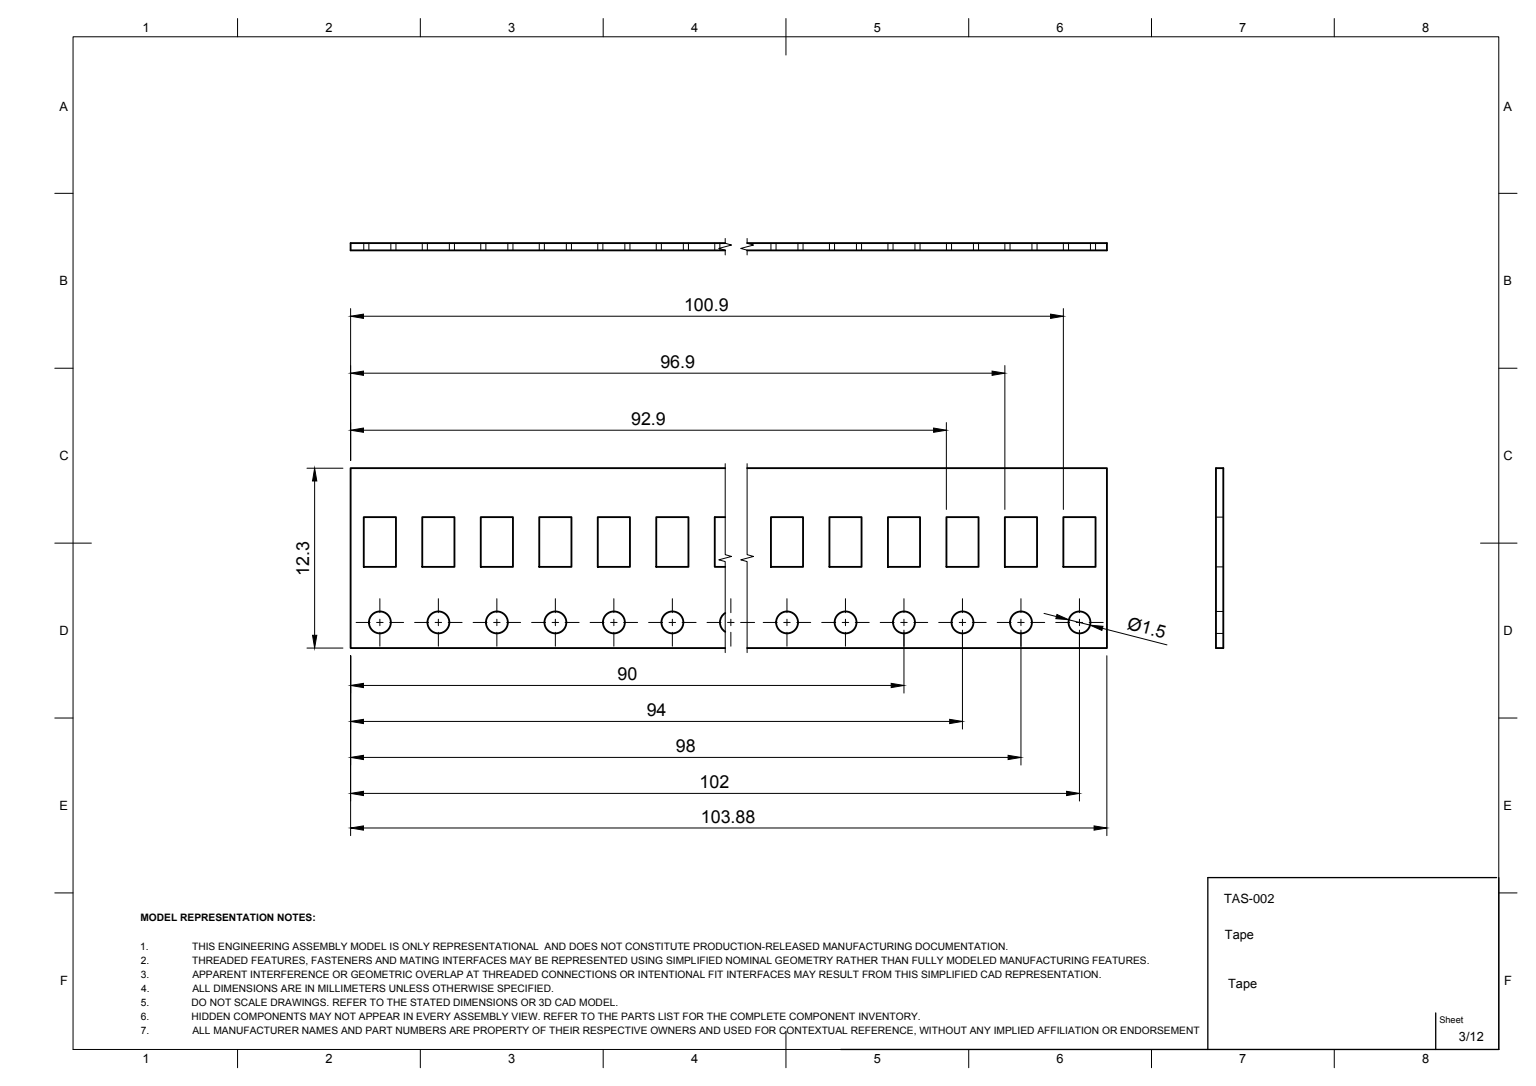
ISO-10303-21;
HEADER;
/* Generated by software containing ST-Developer
 * from STEP Tools, Inc. (www.steptools.com) 
 */

FILE_DESCRIPTION(
/* description */ ('STEP AP214'),
/* implementation_level */ '2;1');

FILE_NAME(
/* name */ 'Tape.step',
/* time_stamp */ '2026-11-04T19:38:14-08:00',
/* author */ (''),
/* organization */ (''),
/* preprocessor_version */ 'ST-DEVELOPER v20.2',
/* originating_system */ 'Autodesk Translation Framework v15.17.0.0',
/* authorisation */ '');

FILE_SCHEMA (('AUTOMOTIVE_DESIGN { 1 0 10303 214 3 1 1 }'));
ENDSEC;

DATA;
#10=MECHANICAL_DESIGN_GEOMETRIC_PRESENTATION_REPRESENTATION('',(#470),#36668);
#450=SHAPE_REPRESENTATION_RELATIONSHIP('SRR','None',#36706,#460);
#460=ADVANCED_BREP_SHAPE_REPRESENTATION('',(#480),#36658);
#470=STYLED_ITEM('',(#36765),#480);
#480=MANIFOLD_SOLID_BREP('Body1',#17793);
#489=CYLINDRICAL_SURFACE('',#17972,0.750000000000001);
#490=CYLINDRICAL_SURFACE('',#17973,0.750000000000001);
#491=CYLINDRICAL_SURFACE('',#17974,0.75);
#492=CYLINDRICAL_SURFACE('',#17975,0.75);
#493=CYLINDRICAL_SURFACE('',#17976,0.75);
#494=CYLINDRICAL_SURFACE('',#17977,0.75);
#495=CYLINDRICAL_SURFACE('',#17978,0.750000000000001);
#496=CYLINDRICAL_SURFACE('',#17979,0.750000000000001);
#497=CYLINDRICAL_SURFACE('',#17980,0.750000000000001);
#498=CYLINDRICAL_SURFACE('',#17981,0.750000000000001);
#499=CYLINDRICAL_SURFACE('',#17982,0.750000000000001);
#500=CYLINDRICAL_SURFACE('',#17983,0.750000000000001);
#501=CYLINDRICAL_SURFACE('',#17984,0.750000000000001);
#502=CYLINDRICAL_SURFACE('',#17985,0.750000000000001);
#503=CYLINDRICAL_SURFACE('',#17986,0.750000000000001);
#504=CYLINDRICAL_SURFACE('',#17987,0.750000000000001);
#505=CYLINDRICAL_SURFACE('',#17988,0.750000000000001);
#506=CYLINDRICAL_SURFACE('',#17989,0.750000000000001);
#507=CYLINDRICAL_SURFACE('',#17990,0.750000000000001);
#508=CYLINDRICAL_SURFACE('',#17991,0.750000000000001);
#509=CYLINDRICAL_SURFACE('',#17992,0.750000000000001);
#510=CYLINDRICAL_SURFACE('',#17993,0.750000000000001);
#511=CYLINDRICAL_SURFACE('',#17994,0.750000000000001);
#512=CYLINDRICAL_SURFACE('',#17995,0.750000000000001);
#513=CYLINDRICAL_SURFACE('',#17996,0.750000000000001);
#514=CYLINDRICAL_SURFACE('',#17997,0.750000000000001);
#776=FACE_BOUND('',#2459,.T.);
#777=FACE_BOUND('',#2460,.T.);
#778=FACE_BOUND('',#2461,.T.);
#779=FACE_BOUND('',#2462,.T.);
#780=FACE_BOUND('',#2463,.T.);
#781=FACE_BOUND('',#2464,.T.);
#782=FACE_BOUND('',#2465,.T.);
#783=FACE_BOUND('',#2466,.T.);
#784=FACE_BOUND('',#2467,.T.);
#785=FACE_BOUND('',#2468,.T.);
#786=FACE_BOUND('',#2469,.T.);
#787=FACE_BOUND('',#2470,.T.);
#788=FACE_BOUND('',#2471,.T.);
#789=FACE_BOUND('',#2472,.T.);
#790=FACE_BOUND('',#2473,.T.);
#791=FACE_BOUND('',#2474,.T.);
#792=FACE_BOUND('',#2475,.T.);
#793=FACE_BOUND('',#2476,.T.);
#794=FACE_BOUND('',#2477,.T.);
#795=FACE_BOUND('',#2478,.T.);
#796=FACE_BOUND('',#2479,.T.);
#797=FACE_BOUND('',#2480,.T.);
#798=FACE_BOUND('',#2481,.T.);
#799=FACE_BOUND('',#2482,.T.);
#800=FACE_BOUND('',#2483,.T.);
#801=FACE_BOUND('',#2484,.T.);
#802=FACE_BOUND('',#2485,.T.);
#803=FACE_BOUND('',#2486,.T.);
#804=FACE_BOUND('',#2487,.T.);
#805=FACE_BOUND('',#2488,.T.);
#806=FACE_BOUND('',#2489,.T.);
#807=FACE_BOUND('',#2490,.T.);
#808=FACE_BOUND('',#2491,.T.);
#809=FACE_BOUND('',#2492,.T.);
#810=FACE_BOUND('',#2493,.T.);
#811=FACE_BOUND('',#2494,.T.);
#812=FACE_BOUND('',#2495,.T.);
#813=FACE_BOUND('',#2496,.T.);
#814=FACE_BOUND('',#2497,.T.);
#815=FACE_BOUND('',#2498,.T.);
#816=FACE_BOUND('',#2499,.T.);
#817=FACE_BOUND('',#2500,.T.);
#818=FACE_BOUND('',#2501,.T.);
#819=FACE_BOUND('',#2502,.T.);
#820=FACE_BOUND('',#2503,.T.);
#821=FACE_BOUND('',#2504,.T.);
#822=FACE_BOUND('',#2505,.T.);
#823=FACE_BOUND('',#2506,.T.);
#824=FACE_BOUND('',#2507,.T.);
#825=FACE_BOUND('',#2508,.T.);
#826=FACE_BOUND('',#2509,.T.);
#827=FACE_BOUND('',#2510,.T.);
#828=FACE_BOUND('',#2512,.T.);
#829=FACE_BOUND('',#2513,.T.);
#830=FACE_BOUND('',#2514,.T.);
#831=FACE_BOUND('',#2515,.T.);
#832=FACE_BOUND('',#2516,.T.);
#833=FACE_BOUND('',#2517,.T.);
#834=FACE_BOUND('',#2518,.T.);
#835=FACE_BOUND('',#2519,.T.);
#836=FACE_BOUND('',#2520,.T.);
#837=FACE_BOUND('',#2521,.T.);
#838=FACE_BOUND('',#2522,.T.);
#839=FACE_BOUND('',#2523,.T.);
#840=FACE_BOUND('',#2524,.T.);
#841=FACE_BOUND('',#2525,.T.);
#842=FACE_BOUND('',#2526,.T.);
#843=FACE_BOUND('',#2527,.T.);
#844=FACE_BOUND('',#2528,.T.);
#845=FACE_BOUND('',#2529,.T.);
#846=FACE_BOUND('',#2530,.T.);
#847=FACE_BOUND('',#2531,.T.);
#848=FACE_BOUND('',#2532,.T.);
#849=FACE_BOUND('',#2533,.T.);
#850=FACE_BOUND('',#2534,.T.);
#851=FACE_BOUND('',#2535,.T.);
#852=FACE_BOUND('',#2536,.T.);
#853=FACE_BOUND('',#2537,.T.);
#854=FACE_BOUND('',#2538,.T.);
#855=FACE_BOUND('',#2539,.T.);
#856=FACE_BOUND('',#2540,.T.);
#857=FACE_BOUND('',#2541,.T.);
#858=FACE_BOUND('',#2542,.T.);
#859=FACE_BOUND('',#2543,.T.);
#860=FACE_BOUND('',#2544,.T.);
#861=FACE_BOUND('',#2545,.T.);
#862=FACE_BOUND('',#2546,.T.);
#863=FACE_BOUND('',#2547,.T.);
#864=FACE_BOUND('',#2548,.T.);
#865=FACE_BOUND('',#2549,.T.);
#866=FACE_BOUND('',#2550,.T.);
#867=FACE_BOUND('',#2551,.T.);
#868=FACE_BOUND('',#2552,.T.);
#869=FACE_BOUND('',#2553,.T.);
#870=FACE_BOUND('',#2554,.T.);
#871=FACE_BOUND('',#2555,.T.);
#872=FACE_BOUND('',#2556,.T.);
#873=FACE_BOUND('',#2557,.T.);
#874=FACE_BOUND('',#2558,.T.);
#875=FACE_BOUND('',#2559,.T.);
#876=FACE_BOUND('',#2560,.T.);
#877=FACE_BOUND('',#2561,.T.);
#878=FACE_BOUND('',#2562,.T.);
#879=FACE_BOUND('',#2563,.T.);
#973=CIRCLE('',#17918,0.750000000000001);
#974=CIRCLE('',#17919,0.750000000000001);
#975=CIRCLE('',#17920,0.750000000000001);
#976=CIRCLE('',#17921,0.75);
#977=CIRCLE('',#17922,0.75);
#978=CIRCLE('',#17923,0.75);
#979=CIRCLE('',#17924,0.75);
#980=CIRCLE('',#17925,0.750000000000001);
#981=CIRCLE('',#17926,0.750000000000001);
#982=CIRCLE('',#17927,0.750000000000001);
#983=CIRCLE('',#17928,0.750000000000001);
#984=CIRCLE('',#17929,0.750000000000001);
#985=CIRCLE('',#17930,0.750000000000001);
#986=CIRCLE('',#17931,0.750000000000001);
#987=CIRCLE('',#17932,0.750000000000001);
#988=CIRCLE('',#17933,0.750000000000001);
#989=CIRCLE('',#17934,0.750000000000001);
#990=CIRCLE('',#17935,0.750000000000001);
#991=CIRCLE('',#17936,0.750000000000001);
#992=CIRCLE('',#17937,0.750000000000001);
#993=CIRCLE('',#17938,0.750000000000001);
#994=CIRCLE('',#17939,0.750000000000001);
#995=CIRCLE('',#17940,0.750000000000001);
#996=CIRCLE('',#17941,0.750000000000001);
#997=CIRCLE('',#17942,0.750000000000001);
#998=CIRCLE('',#17943,0.750000000000001);
#999=CIRCLE('',#17945,0.750000000000001);
#1000=CIRCLE('',#17946,0.750000000000001);
#1001=CIRCLE('',#17947,0.750000000000001);
#1002=CIRCLE('',#17948,0.750000000000001);
#1003=CIRCLE('',#17949,0.750000000000001);
#1004=CIRCLE('',#17950,0.750000000000001);
#1005=CIRCLE('',#17951,0.750000000000001);
#1006=CIRCLE('',#17952,0.750000000000001);
#1007=CIRCLE('',#17953,0.750000000000001);
#1008=CIRCLE('',#17954,0.750000000000001);
#1009=CIRCLE('',#17955,0.750000000000001);
#1010=CIRCLE('',#17956,0.750000000000001);
#1011=CIRCLE('',#17957,0.750000000000001);
#1012=CIRCLE('',#17958,0.750000000000001);
#1013=CIRCLE('',#17959,0.750000000000001);
#1014=CIRCLE('',#17960,0.750000000000001);
#1015=CIRCLE('',#17961,0.750000000000001);
#1016=CIRCLE('',#17962,0.750000000000001);
#1017=CIRCLE('',#17963,0.750000000000001);
#1018=CIRCLE('',#17964,0.75);
#1019=CIRCLE('',#17965,0.75);
#1020=CIRCLE('',#17966,0.75);
#1021=CIRCLE('',#17967,0.75);
#1022=CIRCLE('',#17968,0.750000000000001);
#1023=CIRCLE('',#17969,0.750000000000001);
#1024=CIRCLE('',#17970,0.750000000000001);
#1527=FACE_OUTER_BOUND('',#2458,.T.);
#1528=FACE_OUTER_BOUND('',#2511,.T.);
#1529=FACE_OUTER_BOUND('',#2564,.T.);
#1530=FACE_OUTER_BOUND('',#2565,.T.);
#1531=FACE_OUTER_BOUND('',#2566,.T.);
#1532=FACE_OUTER_BOUND('',#2567,.T.);
#1533=FACE_OUTER_BOUND('',#2568,.T.);
#1534=FACE_OUTER_BOUND('',#2569,.T.);
#1535=FACE_OUTER_BOUND('',#2570,.T.);
#1536=FACE_OUTER_BOUND('',#2571,.T.);
#1537=FACE_OUTER_BOUND('',#2572,.T.);
#1538=FACE_OUTER_BOUND('',#2573,.T.);
#1539=FACE_OUTER_BOUND('',#2574,.T.);
#1540=FACE_OUTER_BOUND('',#2575,.T.);
#1541=FACE_OUTER_BOUND('',#2576,.T.);
#1542=FACE_OUTER_BOUND('',#2577,.T.);
#1543=FACE_OUTER_BOUND('',#2578,.T.);
#1544=FACE_OUTER_BOUND('',#2579,.T.);
#1545=FACE_OUTER_BOUND('',#2580,.T.);
#1546=FACE_OUTER_BOUND('',#2581,.T.);
#1547=FACE_OUTER_BOUND('',#2582,.T.);
#1548=FACE_OUTER_BOUND('',#2583,.T.);
#1549=FACE_OUTER_BOUND('',#2584,.T.);
#1550=FACE_OUTER_BOUND('',#2585,.T.);
#1551=FACE_OUTER_BOUND('',#2586,.T.);
#1552=FACE_OUTER_BOUND('',#2587,.T.);
#1553=FACE_OUTER_BOUND('',#2588,.T.);
#1554=FACE_OUTER_BOUND('',#2589,.T.);
#1555=FACE_OUTER_BOUND('',#2590,.T.);
#1556=FACE_OUTER_BOUND('',#2591,.T.);
#1557=FACE_OUTER_BOUND('',#2592,.T.);
#1558=FACE_OUTER_BOUND('',#2593,.T.);
#1559=FACE_OUTER_BOUND('',#2594,.T.);
#1560=FACE_OUTER_BOUND('',#2595,.T.);
#1561=FACE_OUTER_BOUND('',#2596,.T.);
#1562=FACE_OUTER_BOUND('',#2597,.T.);
#1563=FACE_OUTER_BOUND('',#2598,.T.);
#1564=FACE_OUTER_BOUND('',#2599,.T.);
#1565=FACE_OUTER_BOUND('',#2600,.T.);
#1566=FACE_OUTER_BOUND('',#2601,.T.);
#1567=FACE_OUTER_BOUND('',#2602,.T.);
#1568=FACE_OUTER_BOUND('',#2603,.T.);
#1569=FACE_OUTER_BOUND('',#2604,.T.);
#1570=FACE_OUTER_BOUND('',#2605,.T.);
#1571=FACE_OUTER_BOUND('',#2606,.T.);
#1572=FACE_OUTER_BOUND('',#2607,.T.);
#1573=FACE_OUTER_BOUND('',#2608,.T.);
#1574=FACE_OUTER_BOUND('',#2609,.T.);
#1575=FACE_OUTER_BOUND('',#2610,.T.);
#1576=FACE_OUTER_BOUND('',#2611,.T.);
#1577=FACE_OUTER_BOUND('',#2612,.T.);
#1578=FACE_OUTER_BOUND('',#2613,.T.);
#1579=FACE_OUTER_BOUND('',#2614,.T.);
#1580=FACE_OUTER_BOUND('',#2615,.T.);
#1581=FACE_OUTER_BOUND('',#2616,.T.);
#1582=FACE_OUTER_BOUND('',#2617,.T.);
#1583=FACE_OUTER_BOUND('',#2618,.T.);
#1584=FACE_OUTER_BOUND('',#2619,.T.);
#1585=FACE_OUTER_BOUND('',#2620,.T.);
#1586=FACE_OUTER_BOUND('',#2621,.T.);
#1587=FACE_OUTER_BOUND('',#2622,.T.);
#1588=FACE_OUTER_BOUND('',#2623,.T.);
#1589=FACE_OUTER_BOUND('',#2624,.T.);
#1590=FACE_OUTER_BOUND('',#2625,.T.);
#1591=FACE_OUTER_BOUND('',#2626,.T.);
#1592=FACE_OUTER_BOUND('',#2627,.T.);
#1593=FACE_OUTER_BOUND('',#2628,.T.);
#1594=FACE_OUTER_BOUND('',#2629,.T.);
#1595=FACE_OUTER_BOUND('',#2630,.T.);
#1596=FACE_OUTER_BOUND('',#2631,.T.);
#1597=FACE_OUTER_BOUND('',#2632,.T.);
#1598=FACE_OUTER_BOUND('',#2633,.T.);
#1599=FACE_OUTER_BOUND('',#2634,.T.);
#1600=FACE_OUTER_BOUND('',#2635,.T.);
#1601=FACE_OUTER_BOUND('',#2636,.T.);
#1602=FACE_OUTER_BOUND('',#2637,.T.);
#1603=FACE_OUTER_BOUND('',#2638,.T.);
#1604=FACE_OUTER_BOUND('',#2639,.T.);
#1605=FACE_OUTER_BOUND('',#2640,.T.);
#1606=FACE_OUTER_BOUND('',#2641,.T.);
#1607=FACE_OUTER_BOUND('',#2642,.T.);
#1608=FACE_OUTER_BOUND('',#2643,.T.);
#1609=FACE_OUTER_BOUND('',#2644,.T.);
#1610=FACE_OUTER_BOUND('',#2645,.T.);
#1611=FACE_OUTER_BOUND('',#2646,.T.);
#1612=FACE_OUTER_BOUND('',#2647,.T.);
#1613=FACE_OUTER_BOUND('',#2648,.T.);
#1614=FACE_OUTER_BOUND('',#2649,.T.);
#1615=FACE_OUTER_BOUND('',#2650,.T.);
#1616=FACE_OUTER_BOUND('',#2651,.T.);
#1617=FACE_OUTER_BOUND('',#2652,.T.);
#1618=FACE_OUTER_BOUND('',#2653,.T.);
#1619=FACE_OUTER_BOUND('',#2654,.T.);
#1620=FACE_OUTER_BOUND('',#2655,.T.);
#1621=FACE_OUTER_BOUND('',#2656,.T.);
#1622=FACE_OUTER_BOUND('',#2657,.T.);
#1623=FACE_OUTER_BOUND('',#2658,.T.);
#1624=FACE_OUTER_BOUND('',#2659,.T.);
#1625=FACE_OUTER_BOUND('',#2660,.T.);
#1626=FACE_OUTER_BOUND('',#2661,.T.);
#1627=FACE_OUTER_BOUND('',#2662,.T.);
#1628=FACE_OUTER_BOUND('',#2663,.T.);
#1629=FACE_OUTER_BOUND('',#2664,.T.);
#1630=FACE_OUTER_BOUND('',#2665,.T.);
#1631=FACE_OUTER_BOUND('',#2666,.T.);
#1632=FACE_OUTER_BOUND('',#2667,.T.);
#1633=FACE_OUTER_BOUND('',#2668,.T.);
#1634=FACE_OUTER_BOUND('',#2669,.T.);
#1635=FACE_OUTER_BOUND('',#2670,.T.);
#1636=FACE_OUTER_BOUND('',#2671,.T.);
#1637=FACE_OUTER_BOUND('',#2672,.T.);
#1638=FACE_OUTER_BOUND('',#2673,.T.);
#1639=FACE_OUTER_BOUND('',#2674,.T.);
#1640=FACE_OUTER_BOUND('',#2675,.T.);
#1641=FACE_OUTER_BOUND('',#2676,.T.);
#1642=FACE_OUTER_BOUND('',#2677,.T.);
#1643=FACE_OUTER_BOUND('',#2678,.T.);
#1644=FACE_OUTER_BOUND('',#2679,.T.);
#1645=FACE_OUTER_BOUND('',#2680,.T.);
#1646=FACE_OUTER_BOUND('',#2681,.T.);
#1647=FACE_OUTER_BOUND('',#2682,.T.);
#1648=FACE_OUTER_BOUND('',#2683,.T.);
#1649=FACE_OUTER_BOUND('',#2684,.T.);
#1650=FACE_OUTER_BOUND('',#2685,.T.);
#1651=FACE_OUTER_BOUND('',#2686,.T.);
#1652=FACE_OUTER_BOUND('',#2687,.T.);
#1653=FACE_OUTER_BOUND('',#2688,.T.);
#1654=FACE_OUTER_BOUND('',#2689,.T.);
#1655=FACE_OUTER_BOUND('',#2690,.T.);
#1656=FACE_OUTER_BOUND('',#2691,.T.);
#1657=FACE_OUTER_BOUND('',#2692,.T.);
#1658=FACE_OUTER_BOUND('',#2693,.T.);
#1659=FACE_OUTER_BOUND('',#2694,.T.);
#1660=FACE_OUTER_BOUND('',#2695,.T.);
#1661=FACE_OUTER_BOUND('',#2696,.T.);
#1662=FACE_OUTER_BOUND('',#2697,.T.);
#2458=EDGE_LOOP('',(#11214,#11215,#11216,#11217));
#2459=EDGE_LOOP('',(#11218));
#2460=EDGE_LOOP('',(#11219));
#2461=EDGE_LOOP('',(#11220));
#2462=EDGE_LOOP('',(#11221));
#2463=EDGE_LOOP('',(#11222));
#2464=EDGE_LOOP('',(#11223));
#2465=EDGE_LOOP('',(#11224));
#2466=EDGE_LOOP('',(#11225));
#2467=EDGE_LOOP('',(#11226));
#2468=EDGE_LOOP('',(#11227));
#2469=EDGE_LOOP('',(#11228));
#2470=EDGE_LOOP('',(#11229));
#2471=EDGE_LOOP('',(#11230));
#2472=EDGE_LOOP('',(#11231));
#2473=EDGE_LOOP('',(#11232));
#2474=EDGE_LOOP('',(#11233));
#2475=EDGE_LOOP('',(#11234));
#2476=EDGE_LOOP('',(#11235));
#2477=EDGE_LOOP('',(#11236));
#2478=EDGE_LOOP('',(#11237));
#2479=EDGE_LOOP('',(#11238));
#2480=EDGE_LOOP('',(#11239));
#2481=EDGE_LOOP('',(#11240));
#2482=EDGE_LOOP('',(#11241));
#2483=EDGE_LOOP('',(#11242));
#2484=EDGE_LOOP('',(#11243));
#2485=EDGE_LOOP('',(#11244,#11245,#11246,#11247));
#2486=EDGE_LOOP('',(#11248,#11249,#11250,#11251));
#2487=EDGE_LOOP('',(#11252,#11253,#11254,#11255));
#2488=EDGE_LOOP('',(#11256,#11257,#11258,#11259));
#2489=EDGE_LOOP('',(#11260,#11261,#11262,#11263));
#2490=EDGE_LOOP('',(#11264,#11265,#11266,#11267));
#2491=EDGE_LOOP('',(#11268,#11269,#11270,#11271));
#2492=EDGE_LOOP('',(#11272,#11273,#11274,#11275));
#2493=EDGE_LOOP('',(#11276,#11277,#11278,#11279));
#2494=EDGE_LOOP('',(#11280,#11281,#11282,#11283));
#2495=EDGE_LOOP('',(#11284,#11285,#11286,#11287));
#2496=EDGE_LOOP('',(#11288,#11289,#11290,#11291));
#2497=EDGE_LOOP('',(#11292,#11293,#11294,#11295));
#2498=EDGE_LOOP('',(#11296,#11297,#11298,#11299));
#2499=EDGE_LOOP('',(#11300,#11301,#11302,#11303));
#2500=EDGE_LOOP('',(#11304,#11305,#11306,#11307));
#2501=EDGE_LOOP('',(#11308,#11309,#11310,#11311));
#2502=EDGE_LOOP('',(#11312,#11313,#11314,#11315));
#2503=EDGE_LOOP('',(#11316,#11317,#11318,#11319));
#2504=EDGE_LOOP('',(#11320,#11321,#11322,#11323));
#2505=EDGE_LOOP('',(#11324,#11325,#11326,#11327));
#2506=EDGE_LOOP('',(#11328,#11329,#11330,#11331));
#2507=EDGE_LOOP('',(#11332,#11333,#11334,#11335));
#2508=EDGE_LOOP('',(#11336,#11337,#11338,#11339));
#2509=EDGE_LOOP('',(#11340,#11341,#11342,#11343));
#2510=EDGE_LOOP('',(#11344,#11345,#11346,#11347));
#2511=EDGE_LOOP('',(#11348,#11349,#11350,#11351));
#2512=EDGE_LOOP('',(#11352,#11353,#11354,#11355));
#2513=EDGE_LOOP('',(#11356,#11357,#11358,#11359));
#2514=EDGE_LOOP('',(#11360,#11361,#11362,#11363));
#2515=EDGE_LOOP('',(#11364,#11365,#11366,#11367));
#2516=EDGE_LOOP('',(#11368,#11369,#11370,#11371));
#2517=EDGE_LOOP('',(#11372,#11373,#11374,#11375));
#2518=EDGE_LOOP('',(#11376,#11377,#11378,#11379));
#2519=EDGE_LOOP('',(#11380,#11381,#11382,#11383));
#2520=EDGE_LOOP('',(#11384,#11385,#11386,#11387));
#2521=EDGE_LOOP('',(#11388,#11389,#11390,#11391));
#2522=EDGE_LOOP('',(#11392,#11393,#11394,#11395));
#2523=EDGE_LOOP('',(#11396,#11397,#11398,#11399));
#2524=EDGE_LOOP('',(#11400,#11401,#11402,#11403));
#2525=EDGE_LOOP('',(#11404,#11405,#11406,#11407));
#2526=EDGE_LOOP('',(#11408,#11409,#11410,#11411));
#2527=EDGE_LOOP('',(#11412,#11413,#11414,#11415));
#2528=EDGE_LOOP('',(#11416,#11417,#11418,#11419));
#2529=EDGE_LOOP('',(#11420,#11421,#11422,#11423));
#2530=EDGE_LOOP('',(#11424,#11425,#11426,#11427));
#2531=EDGE_LOOP('',(#11428,#11429,#11430,#11431));
#2532=EDGE_LOOP('',(#11432,#11433,#11434,#11435));
#2533=EDGE_LOOP('',(#11436,#11437,#11438,#11439));
#2534=EDGE_LOOP('',(#11440,#11441,#11442,#11443));
#2535=EDGE_LOOP('',(#11444,#11445,#11446,#11447));
#2536=EDGE_LOOP('',(#11448,#11449,#11450,#11451));
#2537=EDGE_LOOP('',(#11452,#11453,#11454,#11455));
#2538=EDGE_LOOP('',(#11456));
#2539=EDGE_LOOP('',(#11457));
#2540=EDGE_LOOP('',(#11458));
#2541=EDGE_LOOP('',(#11459));
#2542=EDGE_LOOP('',(#11460));
#2543=EDGE_LOOP('',(#11461));
#2544=EDGE_LOOP('',(#11462));
#2545=EDGE_LOOP('',(#11463));
#2546=EDGE_LOOP('',(#11464));
#2547=EDGE_LOOP('',(#11465));
#2548=EDGE_LOOP('',(#11466));
#2549=EDGE_LOOP('',(#11467));
#2550=EDGE_LOOP('',(#11468));
#2551=EDGE_LOOP('',(#11469));
#2552=EDGE_LOOP('',(#11470));
#2553=EDGE_LOOP('',(#11471));
#2554=EDGE_LOOP('',(#11472));
#2555=EDGE_LOOP('',(#11473));
#2556=EDGE_LOOP('',(#11474));
#2557=EDGE_LOOP('',(#11475));
#2558=EDGE_LOOP('',(#11476));
#2559=EDGE_LOOP('',(#11477));
#2560=EDGE_LOOP('',(#11478));
#2561=EDGE_LOOP('',(#11479));
#2562=EDGE_LOOP('',(#11480));
#2563=EDGE_LOOP('',(#11481));
#2564=EDGE_LOOP('',(#11482,#11483,#11484,#11485));
#2565=EDGE_LOOP('',(#11486,#11487,#11488,#11489));
#2566=EDGE_LOOP('',(#11490,#11491,#11492,#11493));
#2567=EDGE_LOOP('',(#11494,#11495,#11496,#11497));
#2568=EDGE_LOOP('',(#11498,#11499,#11500,#11501));
#2569=EDGE_LOOP('',(#11502,#11503,#11504,#11505));
#2570=EDGE_LOOP('',(#11506,#11507,#11508,#11509));
#2571=EDGE_LOOP('',(#11510,#11511,#11512,#11513));
#2572=EDGE_LOOP('',(#11514,#11515,#11516,#11517));
#2573=EDGE_LOOP('',(#11518,#11519,#11520,#11521));
#2574=EDGE_LOOP('',(#11522,#11523,#11524,#11525));
#2575=EDGE_LOOP('',(#11526,#11527,#11528,#11529));
#2576=EDGE_LOOP('',(#11530,#11531,#11532,#11533));
#2577=EDGE_LOOP('',(#11534,#11535,#11536,#11537));
#2578=EDGE_LOOP('',(#11538,#11539,#11540,#11541));
#2579=EDGE_LOOP('',(#11542,#11543,#11544,#11545));
#2580=EDGE_LOOP('',(#11546,#11547,#11548,#11549));
#2581=EDGE_LOOP('',(#11550,#11551,#11552,#11553));
#2582=EDGE_LOOP('',(#11554,#11555,#11556,#11557));
#2583=EDGE_LOOP('',(#11558,#11559,#11560,#11561));
#2584=EDGE_LOOP('',(#11562,#11563,#11564,#11565));
#2585=EDGE_LOOP('',(#11566,#11567,#11568,#11569));
#2586=EDGE_LOOP('',(#11570,#11571,#11572,#11573));
#2587=EDGE_LOOP('',(#11574,#11575,#11576,#11577));
#2588=EDGE_LOOP('',(#11578,#11579,#11580,#11581));
#2589=EDGE_LOOP('',(#11582,#11583,#11584,#11585));
#2590=EDGE_LOOP('',(#11586,#11587,#11588,#11589));
#2591=EDGE_LOOP('',(#11590,#11591,#11592,#11593));
#2592=EDGE_LOOP('',(#11594,#11595,#11596,#11597));
#2593=EDGE_LOOP('',(#11598,#11599,#11600,#11601));
#2594=EDGE_LOOP('',(#11602,#11603,#11604,#11605));
#2595=EDGE_LOOP('',(#11606,#11607,#11608,#11609));
#2596=EDGE_LOOP('',(#11610,#11611,#11612,#11613));
#2597=EDGE_LOOP('',(#11614,#11615,#11616,#11617));
#2598=EDGE_LOOP('',(#11618,#11619,#11620,#11621));
#2599=EDGE_LOOP('',(#11622,#11623,#11624,#11625));
#2600=EDGE_LOOP('',(#11626,#11627,#11628,#11629));
#2601=EDGE_LOOP('',(#11630,#11631,#11632,#11633));
#2602=EDGE_LOOP('',(#11634,#11635,#11636,#11637));
#2603=EDGE_LOOP('',(#11638,#11639,#11640,#11641));
#2604=EDGE_LOOP('',(#11642,#11643,#11644,#11645));
#2605=EDGE_LOOP('',(#11646,#11647,#11648,#11649));
#2606=EDGE_LOOP('',(#11650,#11651,#11652,#11653));
#2607=EDGE_LOOP('',(#11654,#11655,#11656,#11657));
#2608=EDGE_LOOP('',(#11658,#11659,#11660,#11661));
#2609=EDGE_LOOP('',(#11662,#11663,#11664,#11665));
#2610=EDGE_LOOP('',(#11666,#11667,#11668,#11669));
#2611=EDGE_LOOP('',(#11670,#11671,#11672,#11673));
#2612=EDGE_LOOP('',(#11674,#11675,#11676,#11677));
#2613=EDGE_LOOP('',(#11678,#11679,#11680,#11681));
#2614=EDGE_LOOP('',(#11682,#11683,#11684,#11685));
#2615=EDGE_LOOP('',(#11686,#11687,#11688,#11689));
#2616=EDGE_LOOP('',(#11690,#11691,#11692,#11693));
#2617=EDGE_LOOP('',(#11694,#11695,#11696,#11697));
#2618=EDGE_LOOP('',(#11698,#11699,#11700,#11701));
#2619=EDGE_LOOP('',(#11702,#11703,#11704,#11705));
#2620=EDGE_LOOP('',(#11706,#11707,#11708,#11709));
#2621=EDGE_LOOP('',(#11710,#11711,#11712,#11713));
#2622=EDGE_LOOP('',(#11714,#11715,#11716,#11717));
#2623=EDGE_LOOP('',(#11718,#11719,#11720,#11721));
#2624=EDGE_LOOP('',(#11722,#11723,#11724,#11725));
#2625=EDGE_LOOP('',(#11726,#11727,#11728,#11729));
#2626=EDGE_LOOP('',(#11730,#11731,#11732,#11733));
#2627=EDGE_LOOP('',(#11734,#11735,#11736,#11737));
#2628=EDGE_LOOP('',(#11738,#11739,#11740,#11741));
#2629=EDGE_LOOP('',(#11742,#11743,#11744,#11745));
#2630=EDGE_LOOP('',(#11746,#11747,#11748,#11749));
#2631=EDGE_LOOP('',(#11750,#11751,#11752,#11753));
#2632=EDGE_LOOP('',(#11754,#11755,#11756,#11757));
#2633=EDGE_LOOP('',(#11758,#11759,#11760,#11761));
#2634=EDGE_LOOP('',(#11762,#11763,#11764,#11765));
#2635=EDGE_LOOP('',(#11766,#11767,#11768,#11769));
#2636=EDGE_LOOP('',(#11770,#11771,#11772,#11773));
#2637=EDGE_LOOP('',(#11774,#11775,#11776,#11777));
#2638=EDGE_LOOP('',(#11778,#11779,#11780,#11781));
#2639=EDGE_LOOP('',(#11782,#11783,#11784,#11785));
#2640=EDGE_LOOP('',(#11786,#11787,#11788,#11789));
#2641=EDGE_LOOP('',(#11790,#11791,#11792,#11793));
#2642=EDGE_LOOP('',(#11794,#11795,#11796,#11797));
#2643=EDGE_LOOP('',(#11798,#11799,#11800,#11801));
#2644=EDGE_LOOP('',(#11802,#11803,#11804,#11805));
#2645=EDGE_LOOP('',(#11806,#11807,#11808,#11809));
#2646=EDGE_LOOP('',(#11810,#11811,#11812,#11813));
#2647=EDGE_LOOP('',(#11814,#11815,#11816,#11817));
#2648=EDGE_LOOP('',(#11818,#11819,#11820,#11821));
#2649=EDGE_LOOP('',(#11822,#11823,#11824,#11825));
#2650=EDGE_LOOP('',(#11826,#11827,#11828,#11829));
#2651=EDGE_LOOP('',(#11830,#11831,#11832,#11833));
#2652=EDGE_LOOP('',(#11834,#11835,#11836,#11837));
#2653=EDGE_LOOP('',(#11838,#11839,#11840,#11841));
#2654=EDGE_LOOP('',(#11842,#11843,#11844,#11845));
#2655=EDGE_LOOP('',(#11846,#11847,#11848,#11849));
#2656=EDGE_LOOP('',(#11850,#11851,#11852,#11853));
#2657=EDGE_LOOP('',(#11854,#11855,#11856,#11857));
#2658=EDGE_LOOP('',(#11858,#11859,#11860,#11861));
#2659=EDGE_LOOP('',(#11862,#11863,#11864,#11865));
#2660=EDGE_LOOP('',(#11866,#11867,#11868,#11869));
#2661=EDGE_LOOP('',(#11870,#11871,#11872,#11873));
#2662=EDGE_LOOP('',(#11874,#11875,#11876,#11877));
#2663=EDGE_LOOP('',(#11878,#11879,#11880,#11881));
#2664=EDGE_LOOP('',(#11882,#11883,#11884,#11885));
#2665=EDGE_LOOP('',(#11886,#11887,#11888,#11889));
#2666=EDGE_LOOP('',(#11890,#11891,#11892,#11893));
#2667=EDGE_LOOP('',(#11894,#11895,#11896,#11897));
#2668=EDGE_LOOP('',(#11898,#11899,#11900,#11901));
#2669=EDGE_LOOP('',(#11902,#11903,#11904,#11905));
#2670=EDGE_LOOP('',(#11906,#11907,#11908,#11909));
#2671=EDGE_LOOP('',(#11910,#11911,#11912,#11913));
#2672=EDGE_LOOP('',(#11914,#11915,#11916,#11917));
#2673=EDGE_LOOP('',(#11918,#11919,#11920,#11921));
#2674=EDGE_LOOP('',(#11922,#11923,#11924,#11925));
#2675=EDGE_LOOP('',(#11926,#11927,#11928,#11929));
#2676=EDGE_LOOP('',(#11930,#11931,#11932,#11933));
#2677=EDGE_LOOP('',(#11934,#11935,#11936,#11937));
#2678=EDGE_LOOP('',(#11938,#11939,#11940,#11941));
#2679=EDGE_LOOP('',(#11942,#11943,#11944,#11945));
#2680=EDGE_LOOP('',(#11946,#11947,#11948,#11949));
#2681=EDGE_LOOP('',(#11950,#11951,#11952,#11953));
#2682=EDGE_LOOP('',(#11954,#11955,#11956,#11957));
#2683=EDGE_LOOP('',(#11958,#11959,#11960,#11961));
#2684=EDGE_LOOP('',(#11962,#11963,#11964,#11965));
#2685=EDGE_LOOP('',(#11966,#11967,#11968,#11969));
#2686=EDGE_LOOP('',(#11970,#11971,#11972,#11973));
#2687=EDGE_LOOP('',(#11974,#11975,#11976,#11977));
#2688=EDGE_LOOP('',(#11978,#11979,#11980,#11981));
#2689=EDGE_LOOP('',(#11982,#11983,#11984,#11985));
#2690=EDGE_LOOP('',(#11986,#11987,#11988,#11989));
#2691=EDGE_LOOP('',(#11990,#11991,#11992,#11993));
#2692=EDGE_LOOP('',(#11994,#11995,#11996,#11997));
#2693=EDGE_LOOP('',(#11998,#11999,#12000,#12001));
#2694=EDGE_LOOP('',(#12002,#12003,#12004,#12005));
#2695=EDGE_LOOP('',(#12006,#12007,#12008,#12009));
#2696=EDGE_LOOP('',(#12010,#12011,#12012,#12013));
#2697=EDGE_LOOP('',(#12014,#12015,#12016,#12017));
#3586=LINE('',#24199,#5296);
#3587=LINE('',#24201,#5297);
#3588=LINE('',#24203,#5298);
#3589=LINE('',#24204,#5299);
#3590=LINE('',#24259,#5300);
#3591=LINE('',#24261,#5301);
#3592=LINE('',#24263,#5302);
#3593=LINE('',#24264,#5303);
#3594=LINE('',#24267,#5304);
#3595=LINE('',#24269,#5305);
#3596=LINE('',#24271,#5306);
#3597=LINE('',#24272,#5307);
#3598=LINE('',#24275,#5308);
#3599=LINE('',#24277,#5309);
#3600=LINE('',#24279,#5310);
#3601=LINE('',#24280,#5311);
#3602=LINE('',#24283,#5312);
#3603=LINE('',#24285,#5313);
#3604=LINE('',#24287,#5314);
#3605=LINE('',#24288,#5315);
#3606=LINE('',#24291,#5316);
#3607=LINE('',#24293,#5317);
#3608=LINE('',#24295,#5318);
#3609=LINE('',#24296,#5319);
#3610=LINE('',#24299,#5320);
#3611=LINE('',#24301,#5321);
#3612=LINE('',#24303,#5322);
#3613=LINE('',#24304,#5323);
#3614=LINE('',#24307,#5324);
#3615=LINE('',#24309,#5325);
#3616=LINE('',#24311,#5326);
#3617=LINE('',#24312,#5327);
#3618=LINE('',#24315,#5328);
#3619=LINE('',#24317,#5329);
#3620=LINE('',#24319,#5330);
#3621=LINE('',#24320,#5331);
#3622=LINE('',#24323,#5332);
#3623=LINE('',#24325,#5333);
#3624=LINE('',#24327,#5334);
#3625=LINE('',#24328,#5335);
#3626=LINE('',#24331,#5336);
#3627=LINE('',#24333,#5337);
#3628=LINE('',#24335,#5338);
#3629=LINE('',#24336,#5339);
#3630=LINE('',#24339,#5340);
#3631=LINE('',#24341,#5341);
#3632=LINE('',#24343,#5342);
#3633=LINE('',#24344,#5343);
#3634=LINE('',#24347,#5344);
#3635=LINE('',#24349,#5345);
#3636=LINE('',#24351,#5346);
#3637=LINE('',#24352,#5347);
#3638=LINE('',#24355,#5348);
#3639=LINE('',#24357,#5349);
#3640=LINE('',#24359,#5350);
#3641=LINE('',#24360,#5351);
#3642=LINE('',#24363,#5352);
#3643=LINE('',#24365,#5353);
#3644=LINE('',#24367,#5354);
#3645=LINE('',#24368,#5355);
#3646=LINE('',#24371,#5356);
#3647=LINE('',#24373,#5357);
#3648=LINE('',#24375,#5358);
#3649=LINE('',#24376,#5359);
#3650=LINE('',#24379,#5360);
#3651=LINE('',#24381,#5361);
#3652=LINE('',#24383,#5362);
#3653=LINE('',#24384,#5363);
#3654=LINE('',#24387,#5364);
#3655=LINE('',#24389,#5365);
#3656=LINE('',#24391,#5366);
#3657=LINE('',#24392,#5367);
#3658=LINE('',#24395,#5368);
#3659=LINE('',#24397,#5369);
#3660=LINE('',#24399,#5370);
#3661=LINE('',#24400,#5371);
#3662=LINE('',#24403,#5372);
#3663=LINE('',#24405,#5373);
#3664=LINE('',#24407,#5374);
#3665=LINE('',#24408,#5375);
#3666=LINE('',#24411,#5376);
#3667=LINE('',#24413,#5377);
#3668=LINE('',#24415,#5378);
#3669=LINE('',#24416,#5379);
#3670=LINE('',#24419,#5380);
#3671=LINE('',#24421,#5381);
#3672=LINE('',#24423,#5382);
#3673=LINE('',#24424,#5383);
#3674=LINE('',#24427,#5384);
#3675=LINE('',#24429,#5385);
#3676=LINE('',#24431,#5386);
#3677=LINE('',#24432,#5387);
#3678=LINE('',#24435,#5388);
#3679=LINE('',#24437,#5389);
#3680=LINE('',#24439,#5390);
#3681=LINE('',#24440,#5391);
#3682=LINE('',#24443,#5392);
#3683=LINE('',#24445,#5393);
#3684=LINE('',#24447,#5394);
#3685=LINE('',#24448,#5395);
#3686=LINE('',#24451,#5396);
#3687=LINE('',#24453,#5397);
#3688=LINE('',#24455,#5398);
#3689=LINE('',#24456,#5399);
#3690=LINE('',#24459,#5400);
#3691=LINE('',#24461,#5401);
#3692=LINE('',#24463,#5402);
#3693=LINE('',#24464,#5403);
#3694=LINE('',#24468,#5404);
#3695=LINE('',#24470,#5405);
#3696=LINE('',#24472,#5406);
#3697=LINE('',#24473,#5407);
#3698=LINE('',#24476,#5408);
#3699=LINE('',#24478,#5409);
#3700=LINE('',#24480,#5410);
#3701=LINE('',#24481,#5411);
#3702=LINE('',#24484,#5412);
#3703=LINE('',#24486,#5413);
#3704=LINE('',#24488,#5414);
#3705=LINE('',#24489,#5415);
#3706=LINE('',#24492,#5416);
#3707=LINE('',#24494,#5417);
#3708=LINE('',#24496,#5418);
#3709=LINE('',#24497,#5419);
#3710=LINE('',#24500,#5420);
#3711=LINE('',#24502,#5421);
#3712=LINE('',#24504,#5422);
#3713=LINE('',#24505,#5423);
#3714=LINE('',#24508,#5424);
#3715=LINE('',#24510,#5425);
#3716=LINE('',#24512,#5426);
#3717=LINE('',#24513,#5427);
#3718=LINE('',#24516,#5428);
#3719=LINE('',#24518,#5429);
#3720=LINE('',#24520,#5430);
#3721=LINE('',#24521,#5431);
#3722=LINE('',#24524,#5432);
#3723=LINE('',#24526,#5433);
#3724=LINE('',#24528,#5434);
#3725=LINE('',#24529,#5435);
#3726=LINE('',#24532,#5436);
#3727=LINE('',#24534,#5437);
#3728=LINE('',#24536,#5438);
#3729=LINE('',#24537,#5439);
#3730=LINE('',#24540,#5440);
#3731=LINE('',#24542,#5441);
#3732=LINE('',#24544,#5442);
#3733=LINE('',#24545,#5443);
#3734=LINE('',#24548,#5444);
#3735=LINE('',#24550,#5445);
#3736=LINE('',#24552,#5446);
#3737=LINE('',#24553,#5447);
#3738=LINE('',#24556,#5448);
#3739=LINE('',#24558,#5449);
#3740=LINE('',#24560,#5450);
#3741=LINE('',#24561,#5451);
#3742=LINE('',#24564,#5452);
#3743=LINE('',#24566,#5453);
#3744=LINE('',#24568,#5454);
#3745=LINE('',#24569,#5455);
#3746=LINE('',#24572,#5456);
#3747=LINE('',#24574,#5457);
#3748=LINE('',#24576,#5458);
#3749=LINE('',#24577,#5459);
#3750=LINE('',#24580,#5460);
#3751=LINE('',#24582,#5461);
#3752=LINE('',#24584,#5462);
#3753=LINE('',#24585,#5463);
#3754=LINE('',#24588,#5464);
#3755=LINE('',#24590,#5465);
#3756=LINE('',#24592,#5466);
#3757=LINE('',#24593,#5467);
#3758=LINE('',#24596,#5468);
#3759=LINE('',#24598,#5469);
#3760=LINE('',#24600,#5470);
#3761=LINE('',#24601,#5471);
#3762=LINE('',#24604,#5472);
#3763=LINE('',#24606,#5473);
#3764=LINE('',#24608,#5474);
#3765=LINE('',#24609,#5475);
#3766=LINE('',#24612,#5476);
#3767=LINE('',#24614,#5477);
#3768=LINE('',#24616,#5478);
#3769=LINE('',#24617,#5479);
#3770=LINE('',#24620,#5480);
#3771=LINE('',#24622,#5481);
#3772=LINE('',#24624,#5482);
#3773=LINE('',#24625,#5483);
#3774=LINE('',#24628,#5484);
#3775=LINE('',#24630,#5485);
#3776=LINE('',#24632,#5486);
#3777=LINE('',#24633,#5487);
#3778=LINE('',#24636,#5488);
#3779=LINE('',#24638,#5489);
#3780=LINE('',#24640,#5490);
#3781=LINE('',#24641,#5491);
#3782=LINE('',#24644,#5492);
#3783=LINE('',#24646,#5493);
#3784=LINE('',#24648,#5494);
#3785=LINE('',#24649,#5495);
#3786=LINE('',#24652,#5496);
#3787=LINE('',#24654,#5497);
#3788=LINE('',#24656,#5498);
#3789=LINE('',#24657,#5499);
#3790=LINE('',#24660,#5500);
#3791=LINE('',#24662,#5501);
#3792=LINE('',#24664,#5502);
#3793=LINE('',#24665,#5503);
#3794=LINE('',#24668,#5504);
#3795=LINE('',#24670,#5505);
#3796=LINE('',#24672,#5506);
#3797=LINE('',#24673,#5507);
#3798=LINE('',#24676,#5508);
#3799=LINE('',#24678,#5509);
#3800=LINE('',#24680,#5510);
#3801=LINE('',#24681,#5511);
#3802=LINE('',#24735,#5512);
#3803=LINE('',#24736,#5513);
#3804=LINE('',#24738,#5514);
#3805=LINE('',#24740,#5515);
#3806=LINE('',#24742,#5516);
#3807=LINE('',#24744,#5517);
#3808=LINE('',#24746,#5518);
#3809=LINE('',#24748,#5519);
#3810=LINE('',#24750,#5520);
#3811=LINE('',#24752,#5521);
#3812=LINE('',#24754,#5522);
#3813=LINE('',#24756,#5523);
#3814=LINE('',#24758,#5524);
#3815=LINE('',#24760,#5525);
#3816=LINE('',#24762,#5526);
#3817=LINE('',#24764,#5527);
#3818=LINE('',#24766,#5528);
#3819=LINE('',#24768,#5529);
#3820=LINE('',#24770,#5530);
#3821=LINE('',#24772,#5531);
#3822=LINE('',#24774,#5532);
#3823=LINE('',#24776,#5533);
#3824=LINE('',#24778,#5534);
#3825=LINE('',#24780,#5535);
#3826=LINE('',#24782,#5536);
#3827=LINE('',#24784,#5537);
#3828=LINE('',#24786,#5538);
#3829=LINE('',#24788,#5539);
#3830=LINE('',#24790,#5540);
#3831=LINE('',#24791,#5541);
#3832=LINE('',#24793,#5542);
#3833=LINE('',#24794,#5543);
#3834=LINE('',#24796,#5544);
#3835=LINE('',#24797,#5545);
#3836=LINE('',#24799,#5546);
#3837=LINE('',#24800,#5547);
#3838=LINE('',#24802,#5548);
#3839=LINE('',#24803,#5549);
#3840=LINE('',#24805,#5550);
#3841=LINE('',#24806,#5551);
#3842=LINE('',#24808,#5552);
#3843=LINE('',#24809,#5553);
#3844=LINE('',#24811,#5554);
#3845=LINE('',#24812,#5555);
#3846=LINE('',#24814,#5556);
#3847=LINE('',#24815,#5557);
#3848=LINE('',#24817,#5558);
#3849=LINE('',#24818,#5559);
#3850=LINE('',#24820,#5560);
#3851=LINE('',#24821,#5561);
#3852=LINE('',#24823,#5562);
#3853=LINE('',#24824,#5563);
#3854=LINE('',#24826,#5564);
#3855=LINE('',#24827,#5565);
#3856=LINE('',#24829,#5566);
#3857=LINE('',#24830,#5567);
#3858=LINE('',#24832,#5568);
#3859=LINE('',#24833,#5569);
#3860=LINE('',#24835,#5570);
#3861=LINE('',#24836,#5571);
#3862=LINE('',#24838,#5572);
#3863=LINE('',#24839,#5573);
#3864=LINE('',#24841,#5574);
#3865=LINE('',#24842,#5575);
#3866=LINE('',#24844,#5576);
#3867=LINE('',#24845,#5577);
#3868=LINE('',#24847,#5578);
#3869=LINE('',#24848,#5579);
#3870=LINE('',#24850,#5580);
#3871=LINE('',#24851,#5581);
#3872=LINE('',#24853,#5582);
#3873=LINE('',#24854,#5583);
#3874=LINE('',#24856,#5584);
#3875=LINE('',#24857,#5585);
#3876=LINE('',#24859,#5586);
#3877=LINE('',#24860,#5587);
#3878=LINE('',#24862,#5588);
#3879=LINE('',#24863,#5589);
#3880=LINE('',#24865,#5590);
#3881=LINE('',#24866,#5591);
#3882=LINE('',#24868,#5592);
#3883=LINE('',#24870,#5593);
#3884=LINE('',#24872,#5594);
#3885=LINE('',#24874,#5595);
#3886=LINE('',#24877,#5596);
#3887=LINE('',#24879,#5597);
#3888=LINE('',#24882,#5598);
#3889=LINE('',#24884,#5599);
#3890=LINE('',#24887,#5600);
#3891=LINE('',#24889,#5601);
#3892=LINE('',#24892,#5602);
#3893=LINE('',#24894,#5603);
#3894=LINE('',#24897,#5604);
#3895=LINE('',#24899,#5605);
#3896=LINE('',#24902,#5606);
#3897=LINE('',#24904,#5607);
#3898=LINE('',#24907,#5608);
#3899=LINE('',#24909,#5609);
#3900=LINE('',#24912,#5610);
#3901=LINE('',#24914,#5611);
#3902=LINE('',#24917,#5612);
#3903=LINE('',#24919,#5613);
#3904=LINE('',#24922,#5614);
#3905=LINE('',#24924,#5615);
#3906=LINE('',#24927,#5616);
#3907=LINE('',#24929,#5617);
#3908=LINE('',#24932,#5618);
#3909=LINE('',#24934,#5619);
#3910=LINE('',#24937,#5620);
#3911=LINE('',#24939,#5621);
#3912=LINE('',#24942,#5622);
#3913=LINE('',#24944,#5623);
#3914=LINE('',#24947,#5624);
#3915=LINE('',#24949,#5625);
#3916=LINE('',#24952,#5626);
#3917=LINE('',#24954,#5627);
#3918=LINE('',#24957,#5628);
#3919=LINE('',#24959,#5629);
#3920=LINE('',#24962,#5630);
#3921=LINE('',#24964,#5631);
#3922=LINE('',#24967,#5632);
#3923=LINE('',#24969,#5633);
#3924=LINE('',#24972,#5634);
#3925=LINE('',#24974,#5635);
#3926=LINE('',#24977,#5636);
#3927=LINE('',#24979,#5637);
#3928=LINE('',#24982,#5638);
#3929=LINE('',#24984,#5639);
#3930=LINE('',#24987,#5640);
#3931=LINE('',#24989,#5641);
#3932=LINE('',#24992,#5642);
#3933=LINE('',#24994,#5643);
#3934=LINE('',#24997,#5644);
#3935=LINE('',#24999,#5645);
#5296=VECTOR('',#19444,1000.);
#5297=VECTOR('',#19445,1000.);
#5298=VECTOR('',#19446,1000.);
#5299=VECTOR('',#19447,1000.);
#5300=VECTOR('',#19500,1000.);
#5301=VECTOR('',#19501,1000.);
#5302=VECTOR('',#19502,1000.);
#5303=VECTOR('',#19503,1000.);
#5304=VECTOR('',#19504,1000.);
#5305=VECTOR('',#19505,1000.);
#5306=VECTOR('',#19506,1000.);
#5307=VECTOR('',#19507,1000.);
#5308=VECTOR('',#19508,1000.);
#5309=VECTOR('',#19509,1000.);
#5310=VECTOR('',#19510,1000.);
#5311=VECTOR('',#19511,1000.);
#5312=VECTOR('',#19512,1000.);
#5313=VECTOR('',#19513,1000.);
#5314=VECTOR('',#19514,1000.);
#5315=VECTOR('',#19515,1000.);
#5316=VECTOR('',#19516,1000.);
#5317=VECTOR('',#19517,1000.);
#5318=VECTOR('',#19518,1000.);
#5319=VECTOR('',#19519,1000.);
#5320=VECTOR('',#19520,1000.);
#5321=VECTOR('',#19521,1000.);
#5322=VECTOR('',#19522,1000.);
#5323=VECTOR('',#19523,1000.);
#5324=VECTOR('',#19524,1000.);
#5325=VECTOR('',#19525,1000.);
#5326=VECTOR('',#19526,1000.);
#5327=VECTOR('',#19527,1000.);
#5328=VECTOR('',#19528,1000.);
#5329=VECTOR('',#19529,1000.);
#5330=VECTOR('',#19530,1000.);
#5331=VECTOR('',#19531,1000.);
#5332=VECTOR('',#19532,1000.);
#5333=VECTOR('',#19533,1000.);
#5334=VECTOR('',#19534,1000.);
#5335=VECTOR('',#19535,1000.);
#5336=VECTOR('',#19536,1000.);
#5337=VECTOR('',#19537,1000.);
#5338=VECTOR('',#19538,1000.);
#5339=VECTOR('',#19539,1000.);
#5340=VECTOR('',#19540,1000.);
#5341=VECTOR('',#19541,1000.);
#5342=VECTOR('',#19542,1000.);
#5343=VECTOR('',#19543,1000.);
#5344=VECTOR('',#19544,1000.);
#5345=VECTOR('',#19545,1000.);
#5346=VECTOR('',#19546,1000.);
#5347=VECTOR('',#19547,1000.);
#5348=VECTOR('',#19548,1000.);
#5349=VECTOR('',#19549,1000.);
#5350=VECTOR('',#19550,1000.);
#5351=VECTOR('',#19551,1000.);
#5352=VECTOR('',#19552,1000.);
#5353=VECTOR('',#19553,1000.);
#5354=VECTOR('',#19554,1000.);
#5355=VECTOR('',#19555,1000.);
#5356=VECTOR('',#19556,1000.);
#5357=VECTOR('',#19557,1000.);
#5358=VECTOR('',#19558,1000.);
#5359=VECTOR('',#19559,1000.);
#5360=VECTOR('',#19560,1000.);
#5361=VECTOR('',#19561,1000.);
#5362=VECTOR('',#19562,1000.);
#5363=VECTOR('',#19563,1000.);
#5364=VECTOR('',#19564,1000.);
#5365=VECTOR('',#19565,1000.);
#5366=VECTOR('',#19566,1000.);
#5367=VECTOR('',#19567,1000.);
#5368=VECTOR('',#19568,1000.);
#5369=VECTOR('',#19569,1000.);
#5370=VECTOR('',#19570,1000.);
#5371=VECTOR('',#19571,1000.);
#5372=VECTOR('',#19572,1000.);
#5373=VECTOR('',#19573,1000.);
#5374=VECTOR('',#19574,1000.);
#5375=VECTOR('',#19575,1000.);
#5376=VECTOR('',#19576,1000.);
#5377=VECTOR('',#19577,1000.);
#5378=VECTOR('',#19578,1000.);
#5379=VECTOR('',#19579,1000.);
#5380=VECTOR('',#19580,1000.);
#5381=VECTOR('',#19581,1000.);
#5382=VECTOR('',#19582,1000.);
#5383=VECTOR('',#19583,1000.);
#5384=VECTOR('',#19584,1000.);
#5385=VECTOR('',#19585,1000.);
#5386=VECTOR('',#19586,1000.);
#5387=VECTOR('',#19587,1000.);
#5388=VECTOR('',#19588,1000.);
#5389=VECTOR('',#19589,1000.);
#5390=VECTOR('',#19590,1000.);
#5391=VECTOR('',#19591,1000.);
#5392=VECTOR('',#19592,1000.);
#5393=VECTOR('',#19593,1000.);
#5394=VECTOR('',#19594,1000.);
#5395=VECTOR('',#19595,1000.);
#5396=VECTOR('',#19596,1000.);
#5397=VECTOR('',#19597,1000.);
#5398=VECTOR('',#19598,1000.);
#5399=VECTOR('',#19599,1000.);
#5400=VECTOR('',#19600,1000.);
#5401=VECTOR('',#19601,1000.);
#5402=VECTOR('',#19602,1000.);
#5403=VECTOR('',#19603,1000.);
#5404=VECTOR('',#19606,1000.);
#5405=VECTOR('',#19607,1000.);
#5406=VECTOR('',#19608,1000.);
#5407=VECTOR('',#19609,1000.);
#5408=VECTOR('',#19610,1000.);
#5409=VECTOR('',#19611,1000.);
#5410=VECTOR('',#19612,1000.);
#5411=VECTOR('',#19613,1000.);
#5412=VECTOR('',#19614,1000.);
#5413=VECTOR('',#19615,1000.);
#5414=VECTOR('',#19616,1000.);
#5415=VECTOR('',#19617,1000.);
#5416=VECTOR('',#19618,1000.);
#5417=VECTOR('',#19619,1000.);
#5418=VECTOR('',#19620,1000.);
#5419=VECTOR('',#19621,1000.);
#5420=VECTOR('',#19622,1000.);
#5421=VECTOR('',#19623,1000.);
#5422=VECTOR('',#19624,1000.);
#5423=VECTOR('',#19625,1000.);
#5424=VECTOR('',#19626,1000.);
#5425=VECTOR('',#19627,1000.);
#5426=VECTOR('',#19628,1000.);
#5427=VECTOR('',#19629,1000.);
#5428=VECTOR('',#19630,1000.);
#5429=VECTOR('',#19631,1000.);
#5430=VECTOR('',#19632,1000.);
#5431=VECTOR('',#19633,1000.);
#5432=VECTOR('',#19634,1000.);
#5433=VECTOR('',#19635,1000.);
#5434=VECTOR('',#19636,1000.);
#5435=VECTOR('',#19637,1000.);
#5436=VECTOR('',#19638,1000.);
#5437=VECTOR('',#19639,1000.);
#5438=VECTOR('',#19640,1000.);
#5439=VECTOR('',#19641,1000.);
#5440=VECTOR('',#19642,1000.);
#5441=VECTOR('',#19643,1000.);
#5442=VECTOR('',#19644,1000.);
#5443=VECTOR('',#19645,1000.);
#5444=VECTOR('',#19646,1000.);
#5445=VECTOR('',#19647,1000.);
#5446=VECTOR('',#19648,1000.);
#5447=VECTOR('',#19649,1000.);
#5448=VECTOR('',#19650,1000.);
#5449=VECTOR('',#19651,1000.);
#5450=VECTOR('',#19652,1000.);
#5451=VECTOR('',#19653,1000.);
#5452=VECTOR('',#19654,1000.);
#5453=VECTOR('',#19655,1000.);
#5454=VECTOR('',#19656,1000.);
#5455=VECTOR('',#19657,1000.);
#5456=VECTOR('',#19658,1000.);
#5457=VECTOR('',#19659,1000.);
#5458=VECTOR('',#19660,1000.);
#5459=VECTOR('',#19661,1000.);
#5460=VECTOR('',#19662,1000.);
#5461=VECTOR('',#19663,1000.);
#5462=VECTOR('',#19664,1000.);
#5463=VECTOR('',#19665,1000.);
#5464=VECTOR('',#19666,1000.);
#5465=VECTOR('',#19667,1000.);
#5466=VECTOR('',#19668,1000.);
#5467=VECTOR('',#19669,1000.);
#5468=VECTOR('',#19670,1000.);
#5469=VECTOR('',#19671,1000.);
#5470=VECTOR('',#19672,1000.);
#5471=VECTOR('',#19673,1000.);
#5472=VECTOR('',#19674,1000.);
#5473=VECTOR('',#19675,1000.);
#5474=VECTOR('',#19676,1000.);
#5475=VECTOR('',#19677,1000.);
#5476=VECTOR('',#19678,1000.);
#5477=VECTOR('',#19679,1000.);
#5478=VECTOR('',#19680,1000.);
#5479=VECTOR('',#19681,1000.);
#5480=VECTOR('',#19682,1000.);
#5481=VECTOR('',#19683,1000.);
#5482=VECTOR('',#19684,1000.);
#5483=VECTOR('',#19685,1000.);
#5484=VECTOR('',#19686,1000.);
#5485=VECTOR('',#19687,1000.);
#5486=VECTOR('',#19688,1000.);
#5487=VECTOR('',#19689,1000.);
#5488=VECTOR('',#19690,1000.);
#5489=VECTOR('',#19691,1000.);
#5490=VECTOR('',#19692,1000.);
#5491=VECTOR('',#19693,1000.);
#5492=VECTOR('',#19694,1000.);
#5493=VECTOR('',#19695,1000.);
#5494=VECTOR('',#19696,1000.);
#5495=VECTOR('',#19697,1000.);
#5496=VECTOR('',#19698,1000.);
#5497=VECTOR('',#19699,1000.);
#5498=VECTOR('',#19700,1000.);
#5499=VECTOR('',#19701,1000.);
#5500=VECTOR('',#19702,1000.);
#5501=VECTOR('',#19703,1000.);
#5502=VECTOR('',#19704,1000.);
#5503=VECTOR('',#19705,1000.);
#5504=VECTOR('',#19706,1000.);
#5505=VECTOR('',#19707,1000.);
#5506=VECTOR('',#19708,1000.);
#5507=VECTOR('',#19709,1000.);
#5508=VECTOR('',#19710,1000.);
#5509=VECTOR('',#19711,1000.);
#5510=VECTOR('',#19712,1000.);
#5511=VECTOR('',#19713,1000.);
#5512=VECTOR('',#19768,1000.);
#5513=VECTOR('',#19769,1000.);
#5514=VECTOR('',#19772,0.750000000000001);
#5515=VECTOR('',#19775,0.750000000000001);
#5516=VECTOR('',#19778,0.75);
#5517=VECTOR('',#19781,0.75);
#5518=VECTOR('',#19784,0.75);
#5519=VECTOR('',#19787,0.75);
#5520=VECTOR('',#19790,0.750000000000001);
#5521=VECTOR('',#19793,0.750000000000001);
#5522=VECTOR('',#19796,0.750000000000001);
#5523=VECTOR('',#19799,0.750000000000001);
#5524=VECTOR('',#19802,0.750000000000001);
#5525=VECTOR('',#19805,0.750000000000001);
#5526=VECTOR('',#19808,0.750000000000001);
#5527=VECTOR('',#19811,0.750000000000001);
#5528=VECTOR('',#19814,0.750000000000001);
#5529=VECTOR('',#19817,0.750000000000001);
#5530=VECTOR('',#19820,0.750000000000001);
#5531=VECTOR('',#19823,0.750000000000001);
#5532=VECTOR('',#19826,0.750000000000001);
#5533=VECTOR('',#19829,0.750000000000001);
#5534=VECTOR('',#19832,0.750000000000001);
#5535=VECTOR('',#19835,0.750000000000001);
#5536=VECTOR('',#19838,0.750000000000001);
#5537=VECTOR('',#19841,0.750000000000001);
#5538=VECTOR('',#19844,0.750000000000001);
#5539=VECTOR('',#19847,0.750000000000001);
#5540=VECTOR('',#19850,1000.);
#5541=VECTOR('',#19851,1000.);
#5542=VECTOR('',#19854,1000.);
#5543=VECTOR('',#19855,1000.);
#5544=VECTOR('',#19858,1000.);
#5545=VECTOR('',#19859,1000.);
#5546=VECTOR('',#19862,1000.);
#5547=VECTOR('',#19863,1000.);
#5548=VECTOR('',#19866,1000.);
#5549=VECTOR('',#19867,1000.);
#5550=VECTOR('',#19870,1000.);
#5551=VECTOR('',#19871,1000.);
#5552=VECTOR('',#19874,1000.);
#5553=VECTOR('',#19875,1000.);
#5554=VECTOR('',#19878,1000.);
#5555=VECTOR('',#19879,1000.);
#5556=VECTOR('',#19882,1000.);
#5557=VECTOR('',#19883,1000.);
#5558=VECTOR('',#19886,1000.);
#5559=VECTOR('',#19887,1000.);
#5560=VECTOR('',#19890,1000.);
#5561=VECTOR('',#19891,1000.);
#5562=VECTOR('',#19894,1000.);
#5563=VECTOR('',#19895,1000.);
#5564=VECTOR('',#19898,1000.);
#5565=VECTOR('',#19899,1000.);
#5566=VECTOR('',#19902,1000.);
#5567=VECTOR('',#19903,1000.);
#5568=VECTOR('',#19906,1000.);
#5569=VECTOR('',#19907,1000.);
#5570=VECTOR('',#19910,1000.);
#5571=VECTOR('',#19911,1000.);
#5572=VECTOR('',#19914,1000.);
#5573=VECTOR('',#19915,1000.);
#5574=VECTOR('',#19918,1000.);
#5575=VECTOR('',#19919,1000.);
#5576=VECTOR('',#19922,1000.);
#5577=VECTOR('',#19923,1000.);
#5578=VECTOR('',#19926,1000.);
#5579=VECTOR('',#19927,1000.);
#5580=VECTOR('',#19930,1000.);
#5581=VECTOR('',#19931,1000.);
#5582=VECTOR('',#19934,1000.);
#5583=VECTOR('',#19935,1000.);
#5584=VECTOR('',#19938,1000.);
#5585=VECTOR('',#19939,1000.);
#5586=VECTOR('',#19942,1000.);
#5587=VECTOR('',#19943,1000.);
#5588=VECTOR('',#19946,1000.);
#5589=VECTOR('',#19947,1000.);
#5590=VECTOR('',#19950,1000.);
#5591=VECTOR('',#19951,1000.);
#5592=VECTOR('',#19954,1000.);
#5593=VECTOR('',#19957,1000.);
#5594=VECTOR('',#19960,1000.);
#5595=VECTOR('',#19963,1000.);
#5596=VECTOR('',#19968,1000.);
#5597=VECTOR('',#19971,1000.);
#5598=VECTOR('',#19976,1000.);
#5599=VECTOR('',#19979,1000.);
#5600=VECTOR('',#19984,1000.);
#5601=VECTOR('',#19987,1000.);
#5602=VECTOR('',#19992,1000.);
#5603=VECTOR('',#19995,1000.);
#5604=VECTOR('',#20000,1000.);
#5605=VECTOR('',#20003,1000.);
#5606=VECTOR('',#20008,1000.);
#5607=VECTOR('',#20011,1000.);
#5608=VECTOR('',#20016,1000.);
#5609=VECTOR('',#20019,1000.);
#5610=VECTOR('',#20024,1000.);
#5611=VECTOR('',#20027,1000.);
#5612=VECTOR('',#20032,1000.);
#5613=VECTOR('',#20035,1000.);
#5614=VECTOR('',#20040,1000.);
#5615=VECTOR('',#20043,1000.);
#5616=VECTOR('',#20048,1000.);
#5617=VECTOR('',#20051,1000.);
#5618=VECTOR('',#20056,1000.);
#5619=VECTOR('',#20059,1000.);
#5620=VECTOR('',#20064,1000.);
#5621=VECTOR('',#20067,1000.);
#5622=VECTOR('',#20072,1000.);
#5623=VECTOR('',#20075,1000.);
#5624=VECTOR('',#20080,1000.);
#5625=VECTOR('',#20083,1000.);
#5626=VECTOR('',#20088,1000.);
#5627=VECTOR('',#20091,1000.);
#5628=VECTOR('',#20096,1000.);
#5629=VECTOR('',#20099,1000.);
#5630=VECTOR('',#20104,1000.);
#5631=VECTOR('',#20107,1000.);
#5632=VECTOR('',#20112,1000.);
#5633=VECTOR('',#20115,1000.);
#5634=VECTOR('',#20120,1000.);
#5635=VECTOR('',#20123,1000.);
#5636=VECTOR('',#20128,1000.);
#5637=VECTOR('',#20131,1000.);
#5638=VECTOR('',#20136,1000.);
#5639=VECTOR('',#20139,1000.);
#5640=VECTOR('',#20144,1000.);
#5641=VECTOR('',#20147,1000.);
#5642=VECTOR('',#20152,1000.);
#5643=VECTOR('',#20155,1000.);
#5644=VECTOR('',#20160,1000.);
#5645=VECTOR('',#20163,1000.);
#7006=VERTEX_POINT('',#24197);
#7007=VERTEX_POINT('',#24198);
#7008=VERTEX_POINT('',#24200);
#7009=VERTEX_POINT('',#24202);
#7010=VERTEX_POINT('',#24205);
#7011=VERTEX_POINT('',#24207);
#7012=VERTEX_POINT('',#24209);
#7013=VERTEX_POINT('',#24211);
#7014=VERTEX_POINT('',#24213);
#7015=VERTEX_POINT('',#24215);
#7016=VERTEX_POINT('',#24217);
#7017=VERTEX_POINT('',#24219);
#7018=VERTEX_POINT('',#24221);
#7019=VERTEX_POINT('',#24223);
#7020=VERTEX_POINT('',#24225);
#7021=VERTEX_POINT('',#24227);
#7022=VERTEX_POINT('',#24229);
#7023=VERTEX_POINT('',#24231);
#7024=VERTEX_POINT('',#24233);
#7025=VERTEX_POINT('',#24235);
#7026=VERTEX_POINT('',#24237);
#7027=VERTEX_POINT('',#24239);
#7028=VERTEX_POINT('',#24241);
#7029=VERTEX_POINT('',#24243);
#7030=VERTEX_POINT('',#24245);
#7031=VERTEX_POINT('',#24247);
#7032=VERTEX_POINT('',#24249);
#7033=VERTEX_POINT('',#24251);
#7034=VERTEX_POINT('',#24253);
#7035=VERTEX_POINT('',#24255);
#7036=VERTEX_POINT('',#24257);
#7037=VERTEX_POINT('',#24258);
#7038=VERTEX_POINT('',#24260);
#7039=VERTEX_POINT('',#24262);
#7040=VERTEX_POINT('',#24265);
#7041=VERTEX_POINT('',#24266);
#7042=VERTEX_POINT('',#24268);
#7043=VERTEX_POINT('',#24270);
#7044=VERTEX_POINT('',#24273);
#7045=VERTEX_POINT('',#24274);
#7046=VERTEX_POINT('',#24276);
#7047=VERTEX_POINT('',#24278);
#7048=VERTEX_POINT('',#24281);
#7049=VERTEX_POINT('',#24282);
#7050=VERTEX_POINT('',#24284);
#7051=VERTEX_POINT('',#24286);
#7052=VERTEX_POINT('',#24289);
#7053=VERTEX_POINT('',#24290);
#7054=VERTEX_POINT('',#24292);
#7055=VERTEX_POINT('',#24294);
#7056=VERTEX_POINT('',#24297);
#7057=VERTEX_POINT('',#24298);
#7058=VERTEX_POINT('',#24300);
#7059=VERTEX_POINT('',#24302);
#7060=VERTEX_POINT('',#24305);
#7061=VERTEX_POINT('',#24306);
#7062=VERTEX_POINT('',#24308);
#7063=VERTEX_POINT('',#24310);
#7064=VERTEX_POINT('',#24313);
#7065=VERTEX_POINT('',#24314);
#7066=VERTEX_POINT('',#24316);
#7067=VERTEX_POINT('',#24318);
#7068=VERTEX_POINT('',#24321);
#7069=VERTEX_POINT('',#24322);
#7070=VERTEX_POINT('',#24324);
#7071=VERTEX_POINT('',#24326);
#7072=VERTEX_POINT('',#24329);
#7073=VERTEX_POINT('',#24330);
#7074=VERTEX_POINT('',#24332);
#7075=VERTEX_POINT('',#24334);
#7076=VERTEX_POINT('',#24337);
#7077=VERTEX_POINT('',#24338);
#7078=VERTEX_POINT('',#24340);
#7079=VERTEX_POINT('',#24342);
#7080=VERTEX_POINT('',#24345);
#7081=VERTEX_POINT('',#24346);
#7082=VERTEX_POINT('',#24348);
#7083=VERTEX_POINT('',#24350);
#7084=VERTEX_POINT('',#24353);
#7085=VERTEX_POINT('',#24354);
#7086=VERTEX_POINT('',#24356);
#7087=VERTEX_POINT('',#24358);
#7088=VERTEX_POINT('',#24361);
#7089=VERTEX_POINT('',#24362);
#7090=VERTEX_POINT('',#24364);
#7091=VERTEX_POINT('',#24366);
#7092=VERTEX_POINT('',#24369);
#7093=VERTEX_POINT('',#24370);
#7094=VERTEX_POINT('',#24372);
#7095=VERTEX_POINT('',#24374);
#7096=VERTEX_POINT('',#24377);
#7097=VERTEX_POINT('',#24378);
#7098=VERTEX_POINT('',#24380);
#7099=VERTEX_POINT('',#24382);
#7100=VERTEX_POINT('',#24385);
#7101=VERTEX_POINT('',#24386);
#7102=VERTEX_POINT('',#24388);
#7103=VERTEX_POINT('',#24390);
#7104=VERTEX_POINT('',#24393);
#7105=VERTEX_POINT('',#24394);
#7106=VERTEX_POINT('',#24396);
#7107=VERTEX_POINT('',#24398);
#7108=VERTEX_POINT('',#24401);
#7109=VERTEX_POINT('',#24402);
#7110=VERTEX_POINT('',#24404);
#7111=VERTEX_POINT('',#24406);
#7112=VERTEX_POINT('',#24409);
#7113=VERTEX_POINT('',#24410);
#7114=VERTEX_POINT('',#24412);
#7115=VERTEX_POINT('',#24414);
#7116=VERTEX_POINT('',#24417);
#7117=VERTEX_POINT('',#24418);
#7118=VERTEX_POINT('',#24420);
#7119=VERTEX_POINT('',#24422);
#7120=VERTEX_POINT('',#24425);
#7121=VERTEX_POINT('',#24426);
#7122=VERTEX_POINT('',#24428);
#7123=VERTEX_POINT('',#24430);
#7124=VERTEX_POINT('',#24433);
#7125=VERTEX_POINT('',#24434);
#7126=VERTEX_POINT('',#24436);
#7127=VERTEX_POINT('',#24438);
#7128=VERTEX_POINT('',#24441);
#7129=VERTEX_POINT('',#24442);
#7130=VERTEX_POINT('',#24444);
#7131=VERTEX_POINT('',#24446);
#7132=VERTEX_POINT('',#24449);
#7133=VERTEX_POINT('',#24450);
#7134=VERTEX_POINT('',#24452);
#7135=VERTEX_POINT('',#24454);
#7136=VERTEX_POINT('',#24457);
#7137=VERTEX_POINT('',#24458);
#7138=VERTEX_POINT('',#24460);
#7139=VERTEX_POINT('',#24462);
#7140=VERTEX_POINT('',#24466);
#7141=VERTEX_POINT('',#24467);
#7142=VERTEX_POINT('',#24469);
#7143=VERTEX_POINT('',#24471);
#7144=VERTEX_POINT('',#24474);
#7145=VERTEX_POINT('',#24475);
#7146=VERTEX_POINT('',#24477);
#7147=VERTEX_POINT('',#24479);
#7148=VERTEX_POINT('',#24482);
#7149=VERTEX_POINT('',#24483);
#7150=VERTEX_POINT('',#24485);
#7151=VERTEX_POINT('',#24487);
#7152=VERTEX_POINT('',#24490);
#7153=VERTEX_POINT('',#24491);
#7154=VERTEX_POINT('',#24493);
#7155=VERTEX_POINT('',#24495);
#7156=VERTEX_POINT('',#24498);
#7157=VERTEX_POINT('',#24499);
#7158=VERTEX_POINT('',#24501);
#7159=VERTEX_POINT('',#24503);
#7160=VERTEX_POINT('',#24506);
#7161=VERTEX_POINT('',#24507);
#7162=VERTEX_POINT('',#24509);
#7163=VERTEX_POINT('',#24511);
#7164=VERTEX_POINT('',#24514);
#7165=VERTEX_POINT('',#24515);
#7166=VERTEX_POINT('',#24517);
#7167=VERTEX_POINT('',#24519);
#7168=VERTEX_POINT('',#24522);
#7169=VERTEX_POINT('',#24523);
#7170=VERTEX_POINT('',#24525);
#7171=VERTEX_POINT('',#24527);
#7172=VERTEX_POINT('',#24530);
#7173=VERTEX_POINT('',#24531);
#7174=VERTEX_POINT('',#24533);
#7175=VERTEX_POINT('',#24535);
#7176=VERTEX_POINT('',#24538);
#7177=VERTEX_POINT('',#24539);
#7178=VERTEX_POINT('',#24541);
#7179=VERTEX_POINT('',#24543);
#7180=VERTEX_POINT('',#24546);
#7181=VERTEX_POINT('',#24547);
#7182=VERTEX_POINT('',#24549);
#7183=VERTEX_POINT('',#24551);
#7184=VERTEX_POINT('',#24554);
#7185=VERTEX_POINT('',#24555);
#7186=VERTEX_POINT('',#24557);
#7187=VERTEX_POINT('',#24559);
#7188=VERTEX_POINT('',#24562);
#7189=VERTEX_POINT('',#24563);
#7190=VERTEX_POINT('',#24565);
#7191=VERTEX_POINT('',#24567);
#7192=VERTEX_POINT('',#24570);
#7193=VERTEX_POINT('',#24571);
#7194=VERTEX_POINT('',#24573);
#7195=VERTEX_POINT('',#24575);
#7196=VERTEX_POINT('',#24578);
#7197=VERTEX_POINT('',#24579);
#7198=VERTEX_POINT('',#24581);
#7199=VERTEX_POINT('',#24583);
#7200=VERTEX_POINT('',#24586);
#7201=VERTEX_POINT('',#24587);
#7202=VERTEX_POINT('',#24589);
#7203=VERTEX_POINT('',#24591);
#7204=VERTEX_POINT('',#24594);
#7205=VERTEX_POINT('',#24595);
#7206=VERTEX_POINT('',#24597);
#7207=VERTEX_POINT('',#24599);
#7208=VERTEX_POINT('',#24602);
#7209=VERTEX_POINT('',#24603);
#7210=VERTEX_POINT('',#24605);
#7211=VERTEX_POINT('',#24607);
#7212=VERTEX_POINT('',#24610);
#7213=VERTEX_POINT('',#24611);
#7214=VERTEX_POINT('',#24613);
#7215=VERTEX_POINT('',#24615);
#7216=VERTEX_POINT('',#24618);
#7217=VERTEX_POINT('',#24619);
#7218=VERTEX_POINT('',#24621);
#7219=VERTEX_POINT('',#24623);
#7220=VERTEX_POINT('',#24626);
#7221=VERTEX_POINT('',#24627);
#7222=VERTEX_POINT('',#24629);
#7223=VERTEX_POINT('',#24631);
#7224=VERTEX_POINT('',#24634);
#7225=VERTEX_POINT('',#24635);
#7226=VERTEX_POINT('',#24637);
#7227=VERTEX_POINT('',#24639);
#7228=VERTEX_POINT('',#24642);
#7229=VERTEX_POINT('',#24643);
#7230=VERTEX_POINT('',#24645);
#7231=VERTEX_POINT('',#24647);
#7232=VERTEX_POINT('',#24650);
#7233=VERTEX_POINT('',#24651);
#7234=VERTEX_POINT('',#24653);
#7235=VERTEX_POINT('',#24655);
#7236=VERTEX_POINT('',#24658);
#7237=VERTEX_POINT('',#24659);
#7238=VERTEX_POINT('',#24661);
#7239=VERTEX_POINT('',#24663);
#7240=VERTEX_POINT('',#24666);
#7241=VERTEX_POINT('',#24667);
#7242=VERTEX_POINT('',#24669);
#7243=VERTEX_POINT('',#24671);
#7244=VERTEX_POINT('',#24674);
#7245=VERTEX_POINT('',#24675);
#7246=VERTEX_POINT('',#24677);
#7247=VERTEX_POINT('',#24679);
#7248=VERTEX_POINT('',#24682);
#7249=VERTEX_POINT('',#24684);
#7250=VERTEX_POINT('',#24686);
#7251=VERTEX_POINT('',#24688);
#7252=VERTEX_POINT('',#24690);
#7253=VERTEX_POINT('',#24692);
#7254=VERTEX_POINT('',#24694);
#7255=VERTEX_POINT('',#24696);
#7256=VERTEX_POINT('',#24698);
#7257=VERTEX_POINT('',#24700);
#7258=VERTEX_POINT('',#24702);
#7259=VERTEX_POINT('',#24704);
#7260=VERTEX_POINT('',#24706);
#7261=VERTEX_POINT('',#24708);
#7262=VERTEX_POINT('',#24710);
#7263=VERTEX_POINT('',#24712);
#7264=VERTEX_POINT('',#24714);
#7265=VERTEX_POINT('',#24716);
#7266=VERTEX_POINT('',#24718);
#7267=VERTEX_POINT('',#24720);
#7268=VERTEX_POINT('',#24722);
#7269=VERTEX_POINT('',#24724);
#7270=VERTEX_POINT('',#24726);
#7271=VERTEX_POINT('',#24728);
#7272=VERTEX_POINT('',#24730);
#7273=VERTEX_POINT('',#24732);
#8659=EDGE_CURVE('',#7006,#7007,#3586,.T.);
#8660=EDGE_CURVE('',#7006,#7008,#3587,.T.);
#8661=EDGE_CURVE('',#7009,#7008,#3588,.T.);
#8662=EDGE_CURVE('',#7007,#7009,#3589,.T.);
#8663=EDGE_CURVE('',#7010,#7010,#973,.T.);
#8664=EDGE_CURVE('',#7011,#7011,#974,.T.);
#8665=EDGE_CURVE('',#7012,#7012,#975,.T.);
#8666=EDGE_CURVE('',#7013,#7013,#976,.T.);
#8667=EDGE_CURVE('',#7014,#7014,#977,.T.);
#8668=EDGE_CURVE('',#7015,#7015,#978,.T.);
#8669=EDGE_CURVE('',#7016,#7016,#979,.T.);
#8670=EDGE_CURVE('',#7017,#7017,#980,.T.);
#8671=EDGE_CURVE('',#7018,#7018,#981,.T.);
#8672=EDGE_CURVE('',#7019,#7019,#982,.T.);
#8673=EDGE_CURVE('',#7020,#7020,#983,.T.);
#8674=EDGE_CURVE('',#7021,#7021,#984,.T.);
#8675=EDGE_CURVE('',#7022,#7022,#985,.T.);
#8676=EDGE_CURVE('',#7023,#7023,#986,.T.);
#8677=EDGE_CURVE('',#7024,#7024,#987,.T.);
#8678=EDGE_CURVE('',#7025,#7025,#988,.T.);
#8679=EDGE_CURVE('',#7026,#7026,#989,.T.);
#8680=EDGE_CURVE('',#7027,#7027,#990,.T.);
#8681=EDGE_CURVE('',#7028,#7028,#991,.T.);
#8682=EDGE_CURVE('',#7029,#7029,#992,.T.);
#8683=EDGE_CURVE('',#7030,#7030,#993,.T.);
#8684=EDGE_CURVE('',#7031,#7031,#994,.T.);
#8685=EDGE_CURVE('',#7032,#7032,#995,.T.);
#8686=EDGE_CURVE('',#7033,#7033,#996,.T.);
#8687=EDGE_CURVE('',#7034,#7034,#997,.T.);
#8688=EDGE_CURVE('',#7035,#7035,#998,.T.);
#8689=EDGE_CURVE('',#7036,#7037,#3590,.T.);
#8690=EDGE_CURVE('',#7037,#7038,#3591,.T.);
#8691=EDGE_CURVE('',#7039,#7038,#3592,.T.);
#8692=EDGE_CURVE('',#7036,#7039,#3593,.T.);
#8693=EDGE_CURVE('',#7040,#7041,#3594,.T.);
#8694=EDGE_CURVE('',#7041,#7042,#3595,.T.);
#8695=EDGE_CURVE('',#7043,#7042,#3596,.T.);
#8696=EDGE_CURVE('',#7040,#7043,#3597,.T.);
#8697=EDGE_CURVE('',#7044,#7045,#3598,.T.);
#8698=EDGE_CURVE('',#7045,#7046,#3599,.T.);
#8699=EDGE_CURVE('',#7047,#7046,#3600,.T.);
#8700=EDGE_CURVE('',#7044,#7047,#3601,.T.);
#8701=EDGE_CURVE('',#7048,#7049,#3602,.T.);
#8702=EDGE_CURVE('',#7049,#7050,#3603,.T.);
#8703=EDGE_CURVE('',#7051,#7050,#3604,.T.);
#8704=EDGE_CURVE('',#7048,#7051,#3605,.T.);
#8705=EDGE_CURVE('',#7052,#7053,#3606,.T.);
#8706=EDGE_CURVE('',#7053,#7054,#3607,.T.);
#8707=EDGE_CURVE('',#7055,#7054,#3608,.T.);
#8708=EDGE_CURVE('',#7052,#7055,#3609,.T.);
#8709=EDGE_CURVE('',#7056,#7057,#3610,.T.);
#8710=EDGE_CURVE('',#7057,#7058,#3611,.T.);
#8711=EDGE_CURVE('',#7059,#7058,#3612,.T.);
#8712=EDGE_CURVE('',#7056,#7059,#3613,.T.);
#8713=EDGE_CURVE('',#7060,#7061,#3614,.T.);
#8714=EDGE_CURVE('',#7061,#7062,#3615,.T.);
#8715=EDGE_CURVE('',#7063,#7062,#3616,.T.);
#8716=EDGE_CURVE('',#7060,#7063,#3617,.T.);
#8717=EDGE_CURVE('',#7064,#7065,#3618,.T.);
#8718=EDGE_CURVE('',#7065,#7066,#3619,.T.);
#8719=EDGE_CURVE('',#7067,#7066,#3620,.T.);
#8720=EDGE_CURVE('',#7064,#7067,#3621,.T.);
#8721=EDGE_CURVE('',#7068,#7069,#3622,.T.);
#8722=EDGE_CURVE('',#7069,#7070,#3623,.T.);
#8723=EDGE_CURVE('',#7071,#7070,#3624,.T.);
#8724=EDGE_CURVE('',#7068,#7071,#3625,.T.);
#8725=EDGE_CURVE('',#7072,#7073,#3626,.T.);
#8726=EDGE_CURVE('',#7073,#7074,#3627,.T.);
#8727=EDGE_CURVE('',#7075,#7074,#3628,.T.);
#8728=EDGE_CURVE('',#7072,#7075,#3629,.T.);
#8729=EDGE_CURVE('',#7076,#7077,#3630,.T.);
#8730=EDGE_CURVE('',#7077,#7078,#3631,.T.);
#8731=EDGE_CURVE('',#7079,#7078,#3632,.T.);
#8732=EDGE_CURVE('',#7076,#7079,#3633,.T.);
#8733=EDGE_CURVE('',#7080,#7081,#3634,.T.);
#8734=EDGE_CURVE('',#7081,#7082,#3635,.T.);
#8735=EDGE_CURVE('',#7083,#7082,#3636,.T.);
#8736=EDGE_CURVE('',#7080,#7083,#3637,.T.);
#8737=EDGE_CURVE('',#7084,#7085,#3638,.T.);
#8738=EDGE_CURVE('',#7085,#7086,#3639,.T.);
#8739=EDGE_CURVE('',#7087,#7086,#3640,.T.);
#8740=EDGE_CURVE('',#7084,#7087,#3641,.T.);
#8741=EDGE_CURVE('',#7088,#7089,#3642,.T.);
#8742=EDGE_CURVE('',#7089,#7090,#3643,.T.);
#8743=EDGE_CURVE('',#7091,#7090,#3644,.T.);
#8744=EDGE_CURVE('',#7088,#7091,#3645,.T.);
#8745=EDGE_CURVE('',#7092,#7093,#3646,.T.);
#8746=EDGE_CURVE('',#7093,#7094,#3647,.T.);
#8747=EDGE_CURVE('',#7095,#7094,#3648,.T.);
#8748=EDGE_CURVE('',#7092,#7095,#3649,.T.);
#8749=EDGE_CURVE('',#7096,#7097,#3650,.T.);
#8750=EDGE_CURVE('',#7097,#7098,#3651,.T.);
#8751=EDGE_CURVE('',#7099,#7098,#3652,.T.);
#8752=EDGE_CURVE('',#7096,#7099,#3653,.T.);
#8753=EDGE_CURVE('',#7100,#7101,#3654,.T.);
#8754=EDGE_CURVE('',#7101,#7102,#3655,.T.);
#8755=EDGE_CURVE('',#7103,#7102,#3656,.T.);
#8756=EDGE_CURVE('',#7100,#7103,#3657,.T.);
#8757=EDGE_CURVE('',#7104,#7105,#3658,.T.);
#8758=EDGE_CURVE('',#7105,#7106,#3659,.T.);
#8759=EDGE_CURVE('',#7107,#7106,#3660,.T.);
#8760=EDGE_CURVE('',#7104,#7107,#3661,.T.);
#8761=EDGE_CURVE('',#7108,#7109,#3662,.T.);
#8762=EDGE_CURVE('',#7109,#7110,#3663,.T.);
#8763=EDGE_CURVE('',#7111,#7110,#3664,.T.);
#8764=EDGE_CURVE('',#7108,#7111,#3665,.T.);
#8765=EDGE_CURVE('',#7112,#7113,#3666,.T.);
#8766=EDGE_CURVE('',#7113,#7114,#3667,.T.);
#8767=EDGE_CURVE('',#7115,#7114,#3668,.T.);
#8768=EDGE_CURVE('',#7112,#7115,#3669,.T.);
#8769=EDGE_CURVE('',#7116,#7117,#3670,.T.);
#8770=EDGE_CURVE('',#7117,#7118,#3671,.T.);
#8771=EDGE_CURVE('',#7119,#7118,#3672,.T.);
#8772=EDGE_CURVE('',#7116,#7119,#3673,.T.);
#8773=EDGE_CURVE('',#7120,#7121,#3674,.T.);
#8774=EDGE_CURVE('',#7121,#7122,#3675,.T.);
#8775=EDGE_CURVE('',#7123,#7122,#3676,.T.);
#8776=EDGE_CURVE('',#7120,#7123,#3677,.T.);
#8777=EDGE_CURVE('',#7124,#7125,#3678,.T.);
#8778=EDGE_CURVE('',#7125,#7126,#3679,.T.);
#8779=EDGE_CURVE('',#7127,#7126,#3680,.T.);
#8780=EDGE_CURVE('',#7124,#7127,#3681,.T.);
#8781=EDGE_CURVE('',#7128,#7129,#3682,.T.);
#8782=EDGE_CURVE('',#7129,#7130,#3683,.T.);
#8783=EDGE_CURVE('',#7131,#7130,#3684,.T.);
#8784=EDGE_CURVE('',#7128,#7131,#3685,.T.);
#8785=EDGE_CURVE('',#7132,#7133,#3686,.T.);
#8786=EDGE_CURVE('',#7133,#7134,#3687,.T.);
#8787=EDGE_CURVE('',#7135,#7134,#3688,.T.);
#8788=EDGE_CURVE('',#7132,#7135,#3689,.T.);
#8789=EDGE_CURVE('',#7136,#7137,#3690,.T.);
#8790=EDGE_CURVE('',#7137,#7138,#3691,.T.);
#8791=EDGE_CURVE('',#7139,#7138,#3692,.T.);
#8792=EDGE_CURVE('',#7136,#7139,#3693,.T.);
#8793=EDGE_CURVE('',#7140,#7141,#3694,.T.);
#8794=EDGE_CURVE('',#7140,#7142,#3695,.T.);
#8795=EDGE_CURVE('',#7142,#7143,#3696,.T.);
#8796=EDGE_CURVE('',#7141,#7143,#3697,.T.);
#8797=EDGE_CURVE('',#7144,#7145,#3698,.T.);
#8798=EDGE_CURVE('',#7144,#7146,#3699,.T.);
#8799=EDGE_CURVE('',#7146,#7147,#3700,.T.);
#8800=EDGE_CURVE('',#7145,#7147,#3701,.T.);
#8801=EDGE_CURVE('',#7148,#7149,#3702,.T.);
#8802=EDGE_CURVE('',#7148,#7150,#3703,.T.);
#8803=EDGE_CURVE('',#7150,#7151,#3704,.T.);
#8804=EDGE_CURVE('',#7149,#7151,#3705,.T.);
#8805=EDGE_CURVE('',#7152,#7153,#3706,.T.);
#8806=EDGE_CURVE('',#7152,#7154,#3707,.T.);
#8807=EDGE_CURVE('',#7154,#7155,#3708,.T.);
#8808=EDGE_CURVE('',#7153,#7155,#3709,.T.);
#8809=EDGE_CURVE('',#7156,#7157,#3710,.T.);
#8810=EDGE_CURVE('',#7156,#7158,#3711,.T.);
#8811=EDGE_CURVE('',#7158,#7159,#3712,.T.);
#8812=EDGE_CURVE('',#7157,#7159,#3713,.T.);
#8813=EDGE_CURVE('',#7160,#7161,#3714,.T.);
#8814=EDGE_CURVE('',#7160,#7162,#3715,.T.);
#8815=EDGE_CURVE('',#7162,#7163,#3716,.T.);
#8816=EDGE_CURVE('',#7161,#7163,#3717,.T.);
#8817=EDGE_CURVE('',#7164,#7165,#3718,.T.);
#8818=EDGE_CURVE('',#7164,#7166,#3719,.T.);
#8819=EDGE_CURVE('',#7166,#7167,#3720,.T.);
#8820=EDGE_CURVE('',#7165,#7167,#3721,.T.);
#8821=EDGE_CURVE('',#7168,#7169,#3722,.T.);
#8822=EDGE_CURVE('',#7168,#7170,#3723,.T.);
#8823=EDGE_CURVE('',#7170,#7171,#3724,.T.);
#8824=EDGE_CURVE('',#7169,#7171,#3725,.T.);
#8825=EDGE_CURVE('',#7172,#7173,#3726,.T.);
#8826=EDGE_CURVE('',#7172,#7174,#3727,.T.);
#8827=EDGE_CURVE('',#7174,#7175,#3728,.T.);
#8828=EDGE_CURVE('',#7173,#7175,#3729,.T.);
#8829=EDGE_CURVE('',#7176,#7177,#3730,.T.);
#8830=EDGE_CURVE('',#7176,#7178,#3731,.T.);
#8831=EDGE_CURVE('',#7178,#7179,#3732,.T.);
#8832=EDGE_CURVE('',#7177,#7179,#3733,.T.);
#8833=EDGE_CURVE('',#7180,#7181,#3734,.T.);
#8834=EDGE_CURVE('',#7180,#7182,#3735,.T.);
#8835=EDGE_CURVE('',#7182,#7183,#3736,.T.);
#8836=EDGE_CURVE('',#7181,#7183,#3737,.T.);
#8837=EDGE_CURVE('',#7184,#7185,#3738,.T.);
#8838=EDGE_CURVE('',#7184,#7186,#3739,.T.);
#8839=EDGE_CURVE('',#7186,#7187,#3740,.T.);
#8840=EDGE_CURVE('',#7185,#7187,#3741,.T.);
#8841=EDGE_CURVE('',#7188,#7189,#3742,.T.);
#8842=EDGE_CURVE('',#7188,#7190,#3743,.T.);
#8843=EDGE_CURVE('',#7190,#7191,#3744,.T.);
#8844=EDGE_CURVE('',#7189,#7191,#3745,.T.);
#8845=EDGE_CURVE('',#7192,#7193,#3746,.T.);
#8846=EDGE_CURVE('',#7192,#7194,#3747,.T.);
#8847=EDGE_CURVE('',#7194,#7195,#3748,.T.);
#8848=EDGE_CURVE('',#7193,#7195,#3749,.T.);
#8849=EDGE_CURVE('',#7196,#7197,#3750,.T.);
#8850=EDGE_CURVE('',#7196,#7198,#3751,.T.);
#8851=EDGE_CURVE('',#7198,#7199,#3752,.T.);
#8852=EDGE_CURVE('',#7197,#7199,#3753,.T.);
#8853=EDGE_CURVE('',#7200,#7201,#3754,.T.);
#8854=EDGE_CURVE('',#7200,#7202,#3755,.T.);
#8855=EDGE_CURVE('',#7202,#7203,#3756,.T.);
#8856=EDGE_CURVE('',#7201,#7203,#3757,.T.);
#8857=EDGE_CURVE('',#7204,#7205,#3758,.T.);
#8858=EDGE_CURVE('',#7204,#7206,#3759,.T.);
#8859=EDGE_CURVE('',#7206,#7207,#3760,.T.);
#8860=EDGE_CURVE('',#7205,#7207,#3761,.T.);
#8861=EDGE_CURVE('',#7208,#7209,#3762,.T.);
#8862=EDGE_CURVE('',#7208,#7210,#3763,.T.);
#8863=EDGE_CURVE('',#7210,#7211,#3764,.T.);
#8864=EDGE_CURVE('',#7209,#7211,#3765,.T.);
#8865=EDGE_CURVE('',#7212,#7213,#3766,.T.);
#8866=EDGE_CURVE('',#7212,#7214,#3767,.T.);
#8867=EDGE_CURVE('',#7214,#7215,#3768,.T.);
#8868=EDGE_CURVE('',#7213,#7215,#3769,.T.);
#8869=EDGE_CURVE('',#7216,#7217,#3770,.T.);
#8870=EDGE_CURVE('',#7216,#7218,#3771,.T.);
#8871=EDGE_CURVE('',#7218,#7219,#3772,.T.);
#8872=EDGE_CURVE('',#7217,#7219,#3773,.T.);
#8873=EDGE_CURVE('',#7220,#7221,#3774,.T.);
#8874=EDGE_CURVE('',#7220,#7222,#3775,.T.);
#8875=EDGE_CURVE('',#7222,#7223,#3776,.T.);
#8876=EDGE_CURVE('',#7221,#7223,#3777,.T.);
#8877=EDGE_CURVE('',#7224,#7225,#3778,.T.);
#8878=EDGE_CURVE('',#7224,#7226,#3779,.T.);
#8879=EDGE_CURVE('',#7226,#7227,#3780,.T.);
#8880=EDGE_CURVE('',#7225,#7227,#3781,.T.);
#8881=EDGE_CURVE('',#7228,#7229,#3782,.T.);
#8882=EDGE_CURVE('',#7228,#7230,#3783,.T.);
#8883=EDGE_CURVE('',#7230,#7231,#3784,.T.);
#8884=EDGE_CURVE('',#7229,#7231,#3785,.T.);
#8885=EDGE_CURVE('',#7232,#7233,#3786,.T.);
#8886=EDGE_CURVE('',#7232,#7234,#3787,.T.);
#8887=EDGE_CURVE('',#7234,#7235,#3788,.T.);
#8888=EDGE_CURVE('',#7233,#7235,#3789,.T.);
#8889=EDGE_CURVE('',#7236,#7237,#3790,.T.);
#8890=EDGE_CURVE('',#7236,#7238,#3791,.T.);
#8891=EDGE_CURVE('',#7238,#7239,#3792,.T.);
#8892=EDGE_CURVE('',#7237,#7239,#3793,.T.);
#8893=EDGE_CURVE('',#7240,#7241,#3794,.T.);
#8894=EDGE_CURVE('',#7240,#7242,#3795,.T.);
#8895=EDGE_CURVE('',#7242,#7243,#3796,.T.);
#8896=EDGE_CURVE('',#7241,#7243,#3797,.T.);
#8897=EDGE_CURVE('',#7244,#7245,#3798,.T.);
#8898=EDGE_CURVE('',#7244,#7246,#3799,.T.);
#8899=EDGE_CURVE('',#7246,#7247,#3800,.T.);
#8900=EDGE_CURVE('',#7245,#7247,#3801,.T.);
#8901=EDGE_CURVE('',#7248,#7248,#999,.T.);
#8902=EDGE_CURVE('',#7249,#7249,#1000,.T.);
#8903=EDGE_CURVE('',#7250,#7250,#1001,.T.);
#8904=EDGE_CURVE('',#7251,#7251,#1002,.T.);
#8905=EDGE_CURVE('',#7252,#7252,#1003,.T.);
#8906=EDGE_CURVE('',#7253,#7253,#1004,.T.);
#8907=EDGE_CURVE('',#7254,#7254,#1005,.T.);
#8908=EDGE_CURVE('',#7255,#7255,#1006,.T.);
#8909=EDGE_CURVE('',#7256,#7256,#1007,.T.);
#8910=EDGE_CURVE('',#7257,#7257,#1008,.T.);
#8911=EDGE_CURVE('',#7258,#7258,#1009,.T.);
#8912=EDGE_CURVE('',#7259,#7259,#1010,.T.);
#8913=EDGE_CURVE('',#7260,#7260,#1011,.T.);
#8914=EDGE_CURVE('',#7261,#7261,#1012,.T.);
#8915=EDGE_CURVE('',#7262,#7262,#1013,.T.);
#8916=EDGE_CURVE('',#7263,#7263,#1014,.T.);
#8917=EDGE_CURVE('',#7264,#7264,#1015,.T.);
#8918=EDGE_CURVE('',#7265,#7265,#1016,.T.);
#8919=EDGE_CURVE('',#7266,#7266,#1017,.T.);
#8920=EDGE_CURVE('',#7267,#7267,#1018,.T.);
#8921=EDGE_CURVE('',#7268,#7268,#1019,.T.);
#8922=EDGE_CURVE('',#7269,#7269,#1020,.T.);
#8923=EDGE_CURVE('',#7270,#7270,#1021,.T.);
#8924=EDGE_CURVE('',#7271,#7271,#1022,.T.);
#8925=EDGE_CURVE('',#7272,#7272,#1023,.T.);
#8926=EDGE_CURVE('',#7273,#7273,#1024,.T.);
#8927=EDGE_CURVE('',#7145,#7137,#3802,.T.);
#8928=EDGE_CURVE('',#7147,#7138,#3803,.T.);
#8929=EDGE_CURVE('',#7273,#7010,#3804,.T.);
#8930=EDGE_CURVE('',#7272,#7011,#3805,.T.);
#8931=EDGE_CURVE('',#7271,#7012,#3806,.T.);
#8932=EDGE_CURVE('',#7270,#7013,#3807,.T.);
#8933=EDGE_CURVE('',#7269,#7014,#3808,.T.);
#8934=EDGE_CURVE('',#7268,#7015,#3809,.T.);
#8935=EDGE_CURVE('',#7267,#7016,#3810,.T.);
#8936=EDGE_CURVE('',#7266,#7017,#3811,.T.);
#8937=EDGE_CURVE('',#7265,#7018,#3812,.T.);
#8938=EDGE_CURVE('',#7264,#7019,#3813,.T.);
#8939=EDGE_CURVE('',#7263,#7020,#3814,.T.);
#8940=EDGE_CURVE('',#7262,#7021,#3815,.T.);
#8941=EDGE_CURVE('',#7261,#7022,#3816,.T.);
#8942=EDGE_CURVE('',#7260,#7023,#3817,.T.);
#8943=EDGE_CURVE('',#7259,#7024,#3818,.T.);
#8944=EDGE_CURVE('',#7258,#7025,#3819,.T.);
#8945=EDGE_CURVE('',#7257,#7026,#3820,.T.);
#8946=EDGE_CURVE('',#7256,#7027,#3821,.T.);
#8947=EDGE_CURVE('',#7255,#7028,#3822,.T.);
#8948=EDGE_CURVE('',#7254,#7029,#3823,.T.);
#8949=EDGE_CURVE('',#7253,#7030,#3824,.T.);
#8950=EDGE_CURVE('',#7252,#7031,#3825,.T.);
#8951=EDGE_CURVE('',#7251,#7032,#3826,.T.);
#8952=EDGE_CURVE('',#7250,#7033,#3827,.T.);
#8953=EDGE_CURVE('',#7249,#7034,#3828,.T.);
#8954=EDGE_CURVE('',#7248,#7035,#3829,.T.);
#8955=EDGE_CURVE('',#7245,#7037,#3830,.T.);
#8956=EDGE_CURVE('',#7247,#7038,#3831,.T.);
#8957=EDGE_CURVE('',#7241,#7041,#3832,.T.);
#8958=EDGE_CURVE('',#7243,#7042,#3833,.T.);
#8959=EDGE_CURVE('',#7237,#7045,#3834,.T.);
#8960=EDGE_CURVE('',#7239,#7046,#3835,.T.);
#8961=EDGE_CURVE('',#7233,#7049,#3836,.T.);
#8962=EDGE_CURVE('',#7235,#7050,#3837,.T.);
#8963=EDGE_CURVE('',#7229,#7053,#3838,.T.);
#8964=EDGE_CURVE('',#7231,#7054,#3839,.T.);
#8965=EDGE_CURVE('',#7225,#7057,#3840,.T.);
#8966=EDGE_CURVE('',#7227,#7058,#3841,.T.);
#8967=EDGE_CURVE('',#7221,#7061,#3842,.T.);
#8968=EDGE_CURVE('',#7223,#7062,#3843,.T.);
#8969=EDGE_CURVE('',#7217,#7065,#3844,.T.);
#8970=EDGE_CURVE('',#7219,#7066,#3845,.T.);
#8971=EDGE_CURVE('',#7213,#7069,#3846,.T.);
#8972=EDGE_CURVE('',#7215,#7070,#3847,.T.);
#8973=EDGE_CURVE('',#7209,#7073,#3848,.T.);
#8974=EDGE_CURVE('',#7211,#7074,#3849,.T.);
#8975=EDGE_CURVE('',#7205,#7077,#3850,.T.);
#8976=EDGE_CURVE('',#7207,#7078,#3851,.T.);
#8977=EDGE_CURVE('',#7201,#7081,#3852,.T.);
#8978=EDGE_CURVE('',#7203,#7082,#3853,.T.);
#8979=EDGE_CURVE('',#7197,#7085,#3854,.T.);
#8980=EDGE_CURVE('',#7199,#7086,#3855,.T.);
#8981=EDGE_CURVE('',#7193,#7089,#3856,.T.);
#8982=EDGE_CURVE('',#7195,#7090,#3857,.T.);
#8983=EDGE_CURVE('',#7189,#7093,#3858,.T.);
#8984=EDGE_CURVE('',#7191,#7094,#3859,.T.);
#8985=EDGE_CURVE('',#7185,#7097,#3860,.T.);
#8986=EDGE_CURVE('',#7187,#7098,#3861,.T.);
#8987=EDGE_CURVE('',#7181,#7101,#3862,.T.);
#8988=EDGE_CURVE('',#7183,#7102,#3863,.T.);
#8989=EDGE_CURVE('',#7177,#7105,#3864,.T.);
#8990=EDGE_CURVE('',#7179,#7106,#3865,.T.);
#8991=EDGE_CURVE('',#7173,#7109,#3866,.T.);
#8992=EDGE_CURVE('',#7175,#7110,#3867,.T.);
#8993=EDGE_CURVE('',#7169,#7113,#3868,.T.);
#8994=EDGE_CURVE('',#7171,#7114,#3869,.T.);
#8995=EDGE_CURVE('',#7165,#7117,#3870,.T.);
#8996=EDGE_CURVE('',#7167,#7118,#3871,.T.);
#8997=EDGE_CURVE('',#7161,#7121,#3872,.T.);
#8998=EDGE_CURVE('',#7163,#7122,#3873,.T.);
#8999=EDGE_CURVE('',#7157,#7125,#3874,.T.);
#9000=EDGE_CURVE('',#7159,#7126,#3875,.T.);
#9001=EDGE_CURVE('',#7153,#7129,#3876,.T.);
#9002=EDGE_CURVE('',#7155,#7130,#3877,.T.);
#9003=EDGE_CURVE('',#7149,#7133,#3878,.T.);
#9004=EDGE_CURVE('',#7151,#7134,#3879,.T.);
#9005=EDGE_CURVE('',#7141,#7006,#3880,.T.);
#9006=EDGE_CURVE('',#7143,#7008,#3881,.T.);
#9007=EDGE_CURVE('',#7142,#7009,#3882,.T.);
#9008=EDGE_CURVE('',#7140,#7007,#3883,.T.);
#9009=EDGE_CURVE('',#7246,#7039,#3884,.T.);
#9010=EDGE_CURVE('',#7244,#7036,#3885,.T.);
#9011=EDGE_CURVE('',#7242,#7043,#3886,.T.);
#9012=EDGE_CURVE('',#7240,#7040,#3887,.T.);
#9013=EDGE_CURVE('',#7238,#7047,#3888,.T.);
#9014=EDGE_CURVE('',#7236,#7044,#3889,.T.);
#9015=EDGE_CURVE('',#7234,#7051,#3890,.T.);
#9016=EDGE_CURVE('',#7232,#7048,#3891,.T.);
#9017=EDGE_CURVE('',#7230,#7055,#3892,.T.);
#9018=EDGE_CURVE('',#7228,#7052,#3893,.T.);
#9019=EDGE_CURVE('',#7226,#7059,#3894,.T.);
#9020=EDGE_CURVE('',#7224,#7056,#3895,.T.);
#9021=EDGE_CURVE('',#7222,#7063,#3896,.T.);
#9022=EDGE_CURVE('',#7220,#7060,#3897,.T.);
#9023=EDGE_CURVE('',#7218,#7067,#3898,.T.);
#9024=EDGE_CURVE('',#7216,#7064,#3899,.T.);
#9025=EDGE_CURVE('',#7214,#7071,#3900,.T.);
#9026=EDGE_CURVE('',#7212,#7068,#3901,.T.);
#9027=EDGE_CURVE('',#7210,#7075,#3902,.T.);
#9028=EDGE_CURVE('',#7208,#7072,#3903,.T.);
#9029=EDGE_CURVE('',#7206,#7079,#3904,.T.);
#9030=EDGE_CURVE('',#7204,#7076,#3905,.T.);
#9031=EDGE_CURVE('',#7202,#7083,#3906,.T.);
#9032=EDGE_CURVE('',#7200,#7080,#3907,.T.);
#9033=EDGE_CURVE('',#7198,#7087,#3908,.T.);
#9034=EDGE_CURVE('',#7196,#7084,#3909,.T.);
#9035=EDGE_CURVE('',#7194,#7091,#3910,.T.);
#9036=EDGE_CURVE('',#7192,#7088,#3911,.T.);
#9037=EDGE_CURVE('',#7190,#7095,#3912,.T.);
#9038=EDGE_CURVE('',#7188,#7092,#3913,.T.);
#9039=EDGE_CURVE('',#7186,#7099,#3914,.T.);
#9040=EDGE_CURVE('',#7184,#7096,#3915,.T.);
#9041=EDGE_CURVE('',#7182,#7103,#3916,.T.);
#9042=EDGE_CURVE('',#7180,#7100,#3917,.T.);
#9043=EDGE_CURVE('',#7178,#7107,#3918,.T.);
#9044=EDGE_CURVE('',#7176,#7104,#3919,.T.);
#9045=EDGE_CURVE('',#7174,#7111,#3920,.T.);
#9046=EDGE_CURVE('',#7172,#7108,#3921,.T.);
#9047=EDGE_CURVE('',#7170,#7115,#3922,.T.);
#9048=EDGE_CURVE('',#7168,#7112,#3923,.T.);
#9049=EDGE_CURVE('',#7166,#7119,#3924,.T.);
#9050=EDGE_CURVE('',#7164,#7116,#3925,.T.);
#9051=EDGE_CURVE('',#7162,#7123,#3926,.T.);
#9052=EDGE_CURVE('',#7160,#7120,#3927,.T.);
#9053=EDGE_CURVE('',#7158,#7127,#3928,.T.);
#9054=EDGE_CURVE('',#7156,#7124,#3929,.T.);
#9055=EDGE_CURVE('',#7154,#7131,#3930,.T.);
#9056=EDGE_CURVE('',#7152,#7128,#3931,.T.);
#9057=EDGE_CURVE('',#7150,#7135,#3932,.T.);
#9058=EDGE_CURVE('',#7148,#7132,#3933,.T.);
#9059=EDGE_CURVE('',#7146,#7139,#3934,.T.);
#9060=EDGE_CURVE('',#7144,#7136,#3935,.T.);
#11214=ORIENTED_EDGE('',*,*,#8659,.F.);
#11215=ORIENTED_EDGE('',*,*,#8660,.T.);
#11216=ORIENTED_EDGE('',*,*,#8661,.F.);
#11217=ORIENTED_EDGE('',*,*,#8662,.F.);
#11218=ORIENTED_EDGE('',*,*,#8663,.T.);
#11219=ORIENTED_EDGE('',*,*,#8664,.T.);
#11220=ORIENTED_EDGE('',*,*,#8665,.T.);
#11221=ORIENTED_EDGE('',*,*,#8666,.T.);
#11222=ORIENTED_EDGE('',*,*,#8667,.T.);
#11223=ORIENTED_EDGE('',*,*,#8668,.T.);
#11224=ORIENTED_EDGE('',*,*,#8669,.T.);
#11225=ORIENTED_EDGE('',*,*,#8670,.T.);
#11226=ORIENTED_EDGE('',*,*,#8671,.T.);
#11227=ORIENTED_EDGE('',*,*,#8672,.T.);
#11228=ORIENTED_EDGE('',*,*,#8673,.T.);
#11229=ORIENTED_EDGE('',*,*,#8674,.T.);
#11230=ORIENTED_EDGE('',*,*,#8675,.T.);
#11231=ORIENTED_EDGE('',*,*,#8676,.T.);
#11232=ORIENTED_EDGE('',*,*,#8677,.T.);
#11233=ORIENTED_EDGE('',*,*,#8678,.T.);
#11234=ORIENTED_EDGE('',*,*,#8679,.T.);
#11235=ORIENTED_EDGE('',*,*,#8680,.T.);
#11236=ORIENTED_EDGE('',*,*,#8681,.T.);
#11237=ORIENTED_EDGE('',*,*,#8682,.T.);
#11238=ORIENTED_EDGE('',*,*,#8683,.T.);
#11239=ORIENTED_EDGE('',*,*,#8684,.T.);
#11240=ORIENTED_EDGE('',*,*,#8685,.T.);
#11241=ORIENTED_EDGE('',*,*,#8686,.T.);
#11242=ORIENTED_EDGE('',*,*,#8687,.T.);
#11243=ORIENTED_EDGE('',*,*,#8688,.T.);
#11244=ORIENTED_EDGE('',*,*,#8689,.T.);
#11245=ORIENTED_EDGE('',*,*,#8690,.T.);
#11246=ORIENTED_EDGE('',*,*,#8691,.F.);
#11247=ORIENTED_EDGE('',*,*,#8692,.F.);
#11248=ORIENTED_EDGE('',*,*,#8693,.T.);
#11249=ORIENTED_EDGE('',*,*,#8694,.T.);
#11250=ORIENTED_EDGE('',*,*,#8695,.F.);
#11251=ORIENTED_EDGE('',*,*,#8696,.F.);
#11252=ORIENTED_EDGE('',*,*,#8697,.T.);
#11253=ORIENTED_EDGE('',*,*,#8698,.T.);
#11254=ORIENTED_EDGE('',*,*,#8699,.F.);
#11255=ORIENTED_EDGE('',*,*,#8700,.F.);
#11256=ORIENTED_EDGE('',*,*,#8701,.T.);
#11257=ORIENTED_EDGE('',*,*,#8702,.T.);
#11258=ORIENTED_EDGE('',*,*,#8703,.F.);
#11259=ORIENTED_EDGE('',*,*,#8704,.F.);
#11260=ORIENTED_EDGE('',*,*,#8705,.T.);
#11261=ORIENTED_EDGE('',*,*,#8706,.T.);
#11262=ORIENTED_EDGE('',*,*,#8707,.F.);
#11263=ORIENTED_EDGE('',*,*,#8708,.F.);
#11264=ORIENTED_EDGE('',*,*,#8709,.T.);
#11265=ORIENTED_EDGE('',*,*,#8710,.T.);
#11266=ORIENTED_EDGE('',*,*,#8711,.F.);
#11267=ORIENTED_EDGE('',*,*,#8712,.F.);
#11268=ORIENTED_EDGE('',*,*,#8713,.T.);
#11269=ORIENTED_EDGE('',*,*,#8714,.T.);
#11270=ORIENTED_EDGE('',*,*,#8715,.F.);
#11271=ORIENTED_EDGE('',*,*,#8716,.F.);
#11272=ORIENTED_EDGE('',*,*,#8717,.T.);
#11273=ORIENTED_EDGE('',*,*,#8718,.T.);
#11274=ORIENTED_EDGE('',*,*,#8719,.F.);
#11275=ORIENTED_EDGE('',*,*,#8720,.F.);
#11276=ORIENTED_EDGE('',*,*,#8721,.T.);
#11277=ORIENTED_EDGE('',*,*,#8722,.T.);
#11278=ORIENTED_EDGE('',*,*,#8723,.F.);
#11279=ORIENTED_EDGE('',*,*,#8724,.F.);
#11280=ORIENTED_EDGE('',*,*,#8725,.T.);
#11281=ORIENTED_EDGE('',*,*,#8726,.T.);
#11282=ORIENTED_EDGE('',*,*,#8727,.F.);
#11283=ORIENTED_EDGE('',*,*,#8728,.F.);
#11284=ORIENTED_EDGE('',*,*,#8729,.T.);
#11285=ORIENTED_EDGE('',*,*,#8730,.T.);
#11286=ORIENTED_EDGE('',*,*,#8731,.F.);
#11287=ORIENTED_EDGE('',*,*,#8732,.F.);
#11288=ORIENTED_EDGE('',*,*,#8733,.T.);
#11289=ORIENTED_EDGE('',*,*,#8734,.T.);
#11290=ORIENTED_EDGE('',*,*,#8735,.F.);
#11291=ORIENTED_EDGE('',*,*,#8736,.F.);
#11292=ORIENTED_EDGE('',*,*,#8737,.T.);
#11293=ORIENTED_EDGE('',*,*,#8738,.T.);
#11294=ORIENTED_EDGE('',*,*,#8739,.F.);
#11295=ORIENTED_EDGE('',*,*,#8740,.F.);
#11296=ORIENTED_EDGE('',*,*,#8741,.T.);
#11297=ORIENTED_EDGE('',*,*,#8742,.T.);
#11298=ORIENTED_EDGE('',*,*,#8743,.F.);
#11299=ORIENTED_EDGE('',*,*,#8744,.F.);
#11300=ORIENTED_EDGE('',*,*,#8745,.T.);
#11301=ORIENTED_EDGE('',*,*,#8746,.T.);
#11302=ORIENTED_EDGE('',*,*,#8747,.F.);
#11303=ORIENTED_EDGE('',*,*,#8748,.F.);
#11304=ORIENTED_EDGE('',*,*,#8749,.T.);
#11305=ORIENTED_EDGE('',*,*,#8750,.T.);
#11306=ORIENTED_EDGE('',*,*,#8751,.F.);
#11307=ORIENTED_EDGE('',*,*,#8752,.F.);
#11308=ORIENTED_EDGE('',*,*,#8753,.T.);
#11309=ORIENTED_EDGE('',*,*,#8754,.T.);
#11310=ORIENTED_EDGE('',*,*,#8755,.F.);
#11311=ORIENTED_EDGE('',*,*,#8756,.F.);
#11312=ORIENTED_EDGE('',*,*,#8757,.T.);
#11313=ORIENTED_EDGE('',*,*,#8758,.T.);
#11314=ORIENTED_EDGE('',*,*,#8759,.F.);
#11315=ORIENTED_EDGE('',*,*,#8760,.F.);
#11316=ORIENTED_EDGE('',*,*,#8761,.T.);
#11317=ORIENTED_EDGE('',*,*,#8762,.T.);
#11318=ORIENTED_EDGE('',*,*,#8763,.F.);
#11319=ORIENTED_EDGE('',*,*,#8764,.F.);
#11320=ORIENTED_EDGE('',*,*,#8765,.T.);
#11321=ORIENTED_EDGE('',*,*,#8766,.T.);
#11322=ORIENTED_EDGE('',*,*,#8767,.F.);
#11323=ORIENTED_EDGE('',*,*,#8768,.F.);
#11324=ORIENTED_EDGE('',*,*,#8769,.T.);
#11325=ORIENTED_EDGE('',*,*,#8770,.T.);
#11326=ORIENTED_EDGE('',*,*,#8771,.F.);
#11327=ORIENTED_EDGE('',*,*,#8772,.F.);
#11328=ORIENTED_EDGE('',*,*,#8773,.T.);
#11329=ORIENTED_EDGE('',*,*,#8774,.T.);
#11330=ORIENTED_EDGE('',*,*,#8775,.F.);
#11331=ORIENTED_EDGE('',*,*,#8776,.F.);
#11332=ORIENTED_EDGE('',*,*,#8777,.T.);
#11333=ORIENTED_EDGE('',*,*,#8778,.T.);
#11334=ORIENTED_EDGE('',*,*,#8779,.F.);
#11335=ORIENTED_EDGE('',*,*,#8780,.F.);
#11336=ORIENTED_EDGE('',*,*,#8781,.T.);
#11337=ORIENTED_EDGE('',*,*,#8782,.T.);
#11338=ORIENTED_EDGE('',*,*,#8783,.F.);
#11339=ORIENTED_EDGE('',*,*,#8784,.F.);
#11340=ORIENTED_EDGE('',*,*,#8785,.T.);
#11341=ORIENTED_EDGE('',*,*,#8786,.T.);
#11342=ORIENTED_EDGE('',*,*,#8787,.F.);
#11343=ORIENTED_EDGE('',*,*,#8788,.F.);
#11344=ORIENTED_EDGE('',*,*,#8789,.T.);
#11345=ORIENTED_EDGE('',*,*,#8790,.T.);
#11346=ORIENTED_EDGE('',*,*,#8791,.F.);
#11347=ORIENTED_EDGE('',*,*,#8792,.F.);
#11348=ORIENTED_EDGE('',*,*,#8793,.F.);
#11349=ORIENTED_EDGE('',*,*,#8794,.T.);
#11350=ORIENTED_EDGE('',*,*,#8795,.T.);
#11351=ORIENTED_EDGE('',*,*,#8796,.F.);
#11352=ORIENTED_EDGE('',*,*,#8797,.F.);
#11353=ORIENTED_EDGE('',*,*,#8798,.T.);
#11354=ORIENTED_EDGE('',*,*,#8799,.T.);
#11355=ORIENTED_EDGE('',*,*,#8800,.F.);
#11356=ORIENTED_EDGE('',*,*,#8801,.F.);
#11357=ORIENTED_EDGE('',*,*,#8802,.T.);
#11358=ORIENTED_EDGE('',*,*,#8803,.T.);
#11359=ORIENTED_EDGE('',*,*,#8804,.F.);
#11360=ORIENTED_EDGE('',*,*,#8805,.F.);
#11361=ORIENTED_EDGE('',*,*,#8806,.T.);
#11362=ORIENTED_EDGE('',*,*,#8807,.T.);
#11363=ORIENTED_EDGE('',*,*,#8808,.F.);
#11364=ORIENTED_EDGE('',*,*,#8809,.F.);
#11365=ORIENTED_EDGE('',*,*,#8810,.T.);
#11366=ORIENTED_EDGE('',*,*,#8811,.T.);
#11367=ORIENTED_EDGE('',*,*,#8812,.F.);
#11368=ORIENTED_EDGE('',*,*,#8813,.F.);
#11369=ORIENTED_EDGE('',*,*,#8814,.T.);
#11370=ORIENTED_EDGE('',*,*,#8815,.T.);
#11371=ORIENTED_EDGE('',*,*,#8816,.F.);
#11372=ORIENTED_EDGE('',*,*,#8817,.F.);
#11373=ORIENTED_EDGE('',*,*,#8818,.T.);
#11374=ORIENTED_EDGE('',*,*,#8819,.T.);
#11375=ORIENTED_EDGE('',*,*,#8820,.F.);
#11376=ORIENTED_EDGE('',*,*,#8821,.F.);
#11377=ORIENTED_EDGE('',*,*,#8822,.T.);
#11378=ORIENTED_EDGE('',*,*,#8823,.T.);
#11379=ORIENTED_EDGE('',*,*,#8824,.F.);
#11380=ORIENTED_EDGE('',*,*,#8825,.F.);
#11381=ORIENTED_EDGE('',*,*,#8826,.T.);
#11382=ORIENTED_EDGE('',*,*,#8827,.T.);
#11383=ORIENTED_EDGE('',*,*,#8828,.F.);
#11384=ORIENTED_EDGE('',*,*,#8829,.F.);
#11385=ORIENTED_EDGE('',*,*,#8830,.T.);
#11386=ORIENTED_EDGE('',*,*,#8831,.T.);
#11387=ORIENTED_EDGE('',*,*,#8832,.F.);
#11388=ORIENTED_EDGE('',*,*,#8833,.F.);
#11389=ORIENTED_EDGE('',*,*,#8834,.T.);
#11390=ORIENTED_EDGE('',*,*,#8835,.T.);
#11391=ORIENTED_EDGE('',*,*,#8836,.F.);
#11392=ORIENTED_EDGE('',*,*,#8837,.F.);
#11393=ORIENTED_EDGE('',*,*,#8838,.T.);
#11394=ORIENTED_EDGE('',*,*,#8839,.T.);
#11395=ORIENTED_EDGE('',*,*,#8840,.F.);
#11396=ORIENTED_EDGE('',*,*,#8841,.F.);
#11397=ORIENTED_EDGE('',*,*,#8842,.T.);
#11398=ORIENTED_EDGE('',*,*,#8843,.T.);
#11399=ORIENTED_EDGE('',*,*,#8844,.F.);
#11400=ORIENTED_EDGE('',*,*,#8845,.F.);
#11401=ORIENTED_EDGE('',*,*,#8846,.T.);
#11402=ORIENTED_EDGE('',*,*,#8847,.T.);
#11403=ORIENTED_EDGE('',*,*,#8848,.F.);
#11404=ORIENTED_EDGE('',*,*,#8849,.F.);
#11405=ORIENTED_EDGE('',*,*,#8850,.T.);
#11406=ORIENTED_EDGE('',*,*,#8851,.T.);
#11407=ORIENTED_EDGE('',*,*,#8852,.F.);
#11408=ORIENTED_EDGE('',*,*,#8853,.F.);
#11409=ORIENTED_EDGE('',*,*,#8854,.T.);
#11410=ORIENTED_EDGE('',*,*,#8855,.T.);
#11411=ORIENTED_EDGE('',*,*,#8856,.F.);
#11412=ORIENTED_EDGE('',*,*,#8857,.F.);
#11413=ORIENTED_EDGE('',*,*,#8858,.T.);
#11414=ORIENTED_EDGE('',*,*,#8859,.T.);
#11415=ORIENTED_EDGE('',*,*,#8860,.F.);
#11416=ORIENTED_EDGE('',*,*,#8861,.F.);
#11417=ORIENTED_EDGE('',*,*,#8862,.T.);
#11418=ORIENTED_EDGE('',*,*,#8863,.T.);
#11419=ORIENTED_EDGE('',*,*,#8864,.F.);
#11420=ORIENTED_EDGE('',*,*,#8865,.F.);
#11421=ORIENTED_EDGE('',*,*,#8866,.T.);
#11422=ORIENTED_EDGE('',*,*,#8867,.T.);
#11423=ORIENTED_EDGE('',*,*,#8868,.F.);
#11424=ORIENTED_EDGE('',*,*,#8869,.F.);
#11425=ORIENTED_EDGE('',*,*,#8870,.T.);
#11426=ORIENTED_EDGE('',*,*,#8871,.T.);
#11427=ORIENTED_EDGE('',*,*,#8872,.F.);
#11428=ORIENTED_EDGE('',*,*,#8873,.F.);
#11429=ORIENTED_EDGE('',*,*,#8874,.T.);
#11430=ORIENTED_EDGE('',*,*,#8875,.T.);
#11431=ORIENTED_EDGE('',*,*,#8876,.F.);
#11432=ORIENTED_EDGE('',*,*,#8877,.F.);
#11433=ORIENTED_EDGE('',*,*,#8878,.T.);
#11434=ORIENTED_EDGE('',*,*,#8879,.T.);
#11435=ORIENTED_EDGE('',*,*,#8880,.F.);
#11436=ORIENTED_EDGE('',*,*,#8881,.F.);
#11437=ORIENTED_EDGE('',*,*,#8882,.T.);
#11438=ORIENTED_EDGE('',*,*,#8883,.T.);
#11439=ORIENTED_EDGE('',*,*,#8884,.F.);
#11440=ORIENTED_EDGE('',*,*,#8885,.F.);
#11441=ORIENTED_EDGE('',*,*,#8886,.T.);
#11442=ORIENTED_EDGE('',*,*,#8887,.T.);
#11443=ORIENTED_EDGE('',*,*,#8888,.F.);
#11444=ORIENTED_EDGE('',*,*,#8889,.F.);
#11445=ORIENTED_EDGE('',*,*,#8890,.T.);
#11446=ORIENTED_EDGE('',*,*,#8891,.T.);
#11447=ORIENTED_EDGE('',*,*,#8892,.F.);
#11448=ORIENTED_EDGE('',*,*,#8893,.F.);
#11449=ORIENTED_EDGE('',*,*,#8894,.T.);
#11450=ORIENTED_EDGE('',*,*,#8895,.T.);
#11451=ORIENTED_EDGE('',*,*,#8896,.F.);
#11452=ORIENTED_EDGE('',*,*,#8897,.F.);
#11453=ORIENTED_EDGE('',*,*,#8898,.T.);
#11454=ORIENTED_EDGE('',*,*,#8899,.T.);
#11455=ORIENTED_EDGE('',*,*,#8900,.F.);
#11456=ORIENTED_EDGE('',*,*,#8901,.F.);
#11457=ORIENTED_EDGE('',*,*,#8902,.F.);
#11458=ORIENTED_EDGE('',*,*,#8903,.F.);
#11459=ORIENTED_EDGE('',*,*,#8904,.F.);
#11460=ORIENTED_EDGE('',*,*,#8905,.F.);
#11461=ORIENTED_EDGE('',*,*,#8906,.F.);
#11462=ORIENTED_EDGE('',*,*,#8907,.F.);
#11463=ORIENTED_EDGE('',*,*,#8908,.F.);
#11464=ORIENTED_EDGE('',*,*,#8909,.F.);
#11465=ORIENTED_EDGE('',*,*,#8910,.F.);
#11466=ORIENTED_EDGE('',*,*,#8911,.F.);
#11467=ORIENTED_EDGE('',*,*,#8912,.F.);
#11468=ORIENTED_EDGE('',*,*,#8913,.F.);
#11469=ORIENTED_EDGE('',*,*,#8914,.F.);
#11470=ORIENTED_EDGE('',*,*,#8915,.F.);
#11471=ORIENTED_EDGE('',*,*,#8916,.F.);
#11472=ORIENTED_EDGE('',*,*,#8917,.F.);
#11473=ORIENTED_EDGE('',*,*,#8918,.F.);
#11474=ORIENTED_EDGE('',*,*,#8919,.F.);
#11475=ORIENTED_EDGE('',*,*,#8920,.F.);
#11476=ORIENTED_EDGE('',*,*,#8921,.F.);
#11477=ORIENTED_EDGE('',*,*,#8922,.F.);
#11478=ORIENTED_EDGE('',*,*,#8923,.F.);
#11479=ORIENTED_EDGE('',*,*,#8924,.F.);
#11480=ORIENTED_EDGE('',*,*,#8925,.F.);
#11481=ORIENTED_EDGE('',*,*,#8926,.F.);
#11482=ORIENTED_EDGE('',*,*,#8790,.F.);
#11483=ORIENTED_EDGE('',*,*,#8927,.F.);
#11484=ORIENTED_EDGE('',*,*,#8800,.T.);
#11485=ORIENTED_EDGE('',*,*,#8928,.T.);
#11486=ORIENTED_EDGE('',*,*,#8926,.T.);
#11487=ORIENTED_EDGE('',*,*,#8929,.T.);
#11488=ORIENTED_EDGE('',*,*,#8663,.F.);
#11489=ORIENTED_EDGE('',*,*,#8929,.F.);
#11490=ORIENTED_EDGE('',*,*,#8925,.T.);
#11491=ORIENTED_EDGE('',*,*,#8930,.T.);
#11492=ORIENTED_EDGE('',*,*,#8664,.F.);
#11493=ORIENTED_EDGE('',*,*,#8930,.F.);
#11494=ORIENTED_EDGE('',*,*,#8924,.T.);
#11495=ORIENTED_EDGE('',*,*,#8931,.T.);
#11496=ORIENTED_EDGE('',*,*,#8665,.F.);
#11497=ORIENTED_EDGE('',*,*,#8931,.F.);
#11498=ORIENTED_EDGE('',*,*,#8923,.T.);
#11499=ORIENTED_EDGE('',*,*,#8932,.T.);
#11500=ORIENTED_EDGE('',*,*,#8666,.F.);
#11501=ORIENTED_EDGE('',*,*,#8932,.F.);
#11502=ORIENTED_EDGE('',*,*,#8922,.T.);
#11503=ORIENTED_EDGE('',*,*,#8933,.T.);
#11504=ORIENTED_EDGE('',*,*,#8667,.F.);
#11505=ORIENTED_EDGE('',*,*,#8933,.F.);
#11506=ORIENTED_EDGE('',*,*,#8921,.T.);
#11507=ORIENTED_EDGE('',*,*,#8934,.T.);
#11508=ORIENTED_EDGE('',*,*,#8668,.F.);
#11509=ORIENTED_EDGE('',*,*,#8934,.F.);
#11510=ORIENTED_EDGE('',*,*,#8920,.T.);
#11511=ORIENTED_EDGE('',*,*,#8935,.T.);
#11512=ORIENTED_EDGE('',*,*,#8669,.F.);
#11513=ORIENTED_EDGE('',*,*,#8935,.F.);
#11514=ORIENTED_EDGE('',*,*,#8919,.T.);
#11515=ORIENTED_EDGE('',*,*,#8936,.T.);
#11516=ORIENTED_EDGE('',*,*,#8670,.F.);
#11517=ORIENTED_EDGE('',*,*,#8936,.F.);
#11518=ORIENTED_EDGE('',*,*,#8918,.T.);
#11519=ORIENTED_EDGE('',*,*,#8937,.T.);
#11520=ORIENTED_EDGE('',*,*,#8671,.F.);
#11521=ORIENTED_EDGE('',*,*,#8937,.F.);
#11522=ORIENTED_EDGE('',*,*,#8917,.T.);
#11523=ORIENTED_EDGE('',*,*,#8938,.T.);
#11524=ORIENTED_EDGE('',*,*,#8672,.F.);
#11525=ORIENTED_EDGE('',*,*,#8938,.F.);
#11526=ORIENTED_EDGE('',*,*,#8916,.T.);
#11527=ORIENTED_EDGE('',*,*,#8939,.T.);
#11528=ORIENTED_EDGE('',*,*,#8673,.F.);
#11529=ORIENTED_EDGE('',*,*,#8939,.F.);
#11530=ORIENTED_EDGE('',*,*,#8915,.T.);
#11531=ORIENTED_EDGE('',*,*,#8940,.T.);
#11532=ORIENTED_EDGE('',*,*,#8674,.F.);
#11533=ORIENTED_EDGE('',*,*,#8940,.F.);
#11534=ORIENTED_EDGE('',*,*,#8914,.T.);
#11535=ORIENTED_EDGE('',*,*,#8941,.T.);
#11536=ORIENTED_EDGE('',*,*,#8675,.F.);
#11537=ORIENTED_EDGE('',*,*,#8941,.F.);
#11538=ORIENTED_EDGE('',*,*,#8913,.T.);
#11539=ORIENTED_EDGE('',*,*,#8942,.T.);
#11540=ORIENTED_EDGE('',*,*,#8676,.F.);
#11541=ORIENTED_EDGE('',*,*,#8942,.F.);
#11542=ORIENTED_EDGE('',*,*,#8912,.T.);
#11543=ORIENTED_EDGE('',*,*,#8943,.T.);
#11544=ORIENTED_EDGE('',*,*,#8677,.F.);
#11545=ORIENTED_EDGE('',*,*,#8943,.F.);
#11546=ORIENTED_EDGE('',*,*,#8911,.T.);
#11547=ORIENTED_EDGE('',*,*,#8944,.T.);
#11548=ORIENTED_EDGE('',*,*,#8678,.F.);
#11549=ORIENTED_EDGE('',*,*,#8944,.F.);
#11550=ORIENTED_EDGE('',*,*,#8910,.T.);
#11551=ORIENTED_EDGE('',*,*,#8945,.T.);
#11552=ORIENTED_EDGE('',*,*,#8679,.F.);
#11553=ORIENTED_EDGE('',*,*,#8945,.F.);
#11554=ORIENTED_EDGE('',*,*,#8909,.T.);
#11555=ORIENTED_EDGE('',*,*,#8946,.T.);
#11556=ORIENTED_EDGE('',*,*,#8680,.F.);
#11557=ORIENTED_EDGE('',*,*,#8946,.F.);
#11558=ORIENTED_EDGE('',*,*,#8908,.T.);
#11559=ORIENTED_EDGE('',*,*,#8947,.T.);
#11560=ORIENTED_EDGE('',*,*,#8681,.F.);
#11561=ORIENTED_EDGE('',*,*,#8947,.F.);
#11562=ORIENTED_EDGE('',*,*,#8907,.T.);
#11563=ORIENTED_EDGE('',*,*,#8948,.T.);
#11564=ORIENTED_EDGE('',*,*,#8682,.F.);
#11565=ORIENTED_EDGE('',*,*,#8948,.F.);
#11566=ORIENTED_EDGE('',*,*,#8906,.T.);
#11567=ORIENTED_EDGE('',*,*,#8949,.T.);
#11568=ORIENTED_EDGE('',*,*,#8683,.F.);
#11569=ORIENTED_EDGE('',*,*,#8949,.F.);
#11570=ORIENTED_EDGE('',*,*,#8905,.T.);
#11571=ORIENTED_EDGE('',*,*,#8950,.T.);
#11572=ORIENTED_EDGE('',*,*,#8684,.F.);
#11573=ORIENTED_EDGE('',*,*,#8950,.F.);
#11574=ORIENTED_EDGE('',*,*,#8904,.T.);
#11575=ORIENTED_EDGE('',*,*,#8951,.T.);
#11576=ORIENTED_EDGE('',*,*,#8685,.F.);
#11577=ORIENTED_EDGE('',*,*,#8951,.F.);
#11578=ORIENTED_EDGE('',*,*,#8903,.T.);
#11579=ORIENTED_EDGE('',*,*,#8952,.T.);
#11580=ORIENTED_EDGE('',*,*,#8686,.F.);
#11581=ORIENTED_EDGE('',*,*,#8952,.F.);
#11582=ORIENTED_EDGE('',*,*,#8902,.T.);
#11583=ORIENTED_EDGE('',*,*,#8953,.T.);
#11584=ORIENTED_EDGE('',*,*,#8687,.F.);
#11585=ORIENTED_EDGE('',*,*,#8953,.F.);
#11586=ORIENTED_EDGE('',*,*,#8901,.T.);
#11587=ORIENTED_EDGE('',*,*,#8954,.T.);
#11588=ORIENTED_EDGE('',*,*,#8688,.F.);
#11589=ORIENTED_EDGE('',*,*,#8954,.F.);
#11590=ORIENTED_EDGE('',*,*,#8690,.F.);
#11591=ORIENTED_EDGE('',*,*,#8955,.F.);
#11592=ORIENTED_EDGE('',*,*,#8900,.T.);
#11593=ORIENTED_EDGE('',*,*,#8956,.T.);
#11594=ORIENTED_EDGE('',*,*,#8694,.F.);
#11595=ORIENTED_EDGE('',*,*,#8957,.F.);
#11596=ORIENTED_EDGE('',*,*,#8896,.T.);
#11597=ORIENTED_EDGE('',*,*,#8958,.T.);
#11598=ORIENTED_EDGE('',*,*,#8698,.F.);
#11599=ORIENTED_EDGE('',*,*,#8959,.F.);
#11600=ORIENTED_EDGE('',*,*,#8892,.T.);
#11601=ORIENTED_EDGE('',*,*,#8960,.T.);
#11602=ORIENTED_EDGE('',*,*,#8702,.F.);
#11603=ORIENTED_EDGE('',*,*,#8961,.F.);
#11604=ORIENTED_EDGE('',*,*,#8888,.T.);
#11605=ORIENTED_EDGE('',*,*,#8962,.T.);
#11606=ORIENTED_EDGE('',*,*,#8706,.F.);
#11607=ORIENTED_EDGE('',*,*,#8963,.F.);
#11608=ORIENTED_EDGE('',*,*,#8884,.T.);
#11609=ORIENTED_EDGE('',*,*,#8964,.T.);
#11610=ORIENTED_EDGE('',*,*,#8710,.F.);
#11611=ORIENTED_EDGE('',*,*,#8965,.F.);
#11612=ORIENTED_EDGE('',*,*,#8880,.T.);
#11613=ORIENTED_EDGE('',*,*,#8966,.T.);
#11614=ORIENTED_EDGE('',*,*,#8714,.F.);
#11615=ORIENTED_EDGE('',*,*,#8967,.F.);
#11616=ORIENTED_EDGE('',*,*,#8876,.T.);
#11617=ORIENTED_EDGE('',*,*,#8968,.T.);
#11618=ORIENTED_EDGE('',*,*,#8718,.F.);
#11619=ORIENTED_EDGE('',*,*,#8969,.F.);
#11620=ORIENTED_EDGE('',*,*,#8872,.T.);
#11621=ORIENTED_EDGE('',*,*,#8970,.T.);
#11622=ORIENTED_EDGE('',*,*,#8722,.F.);
#11623=ORIENTED_EDGE('',*,*,#8971,.F.);
#11624=ORIENTED_EDGE('',*,*,#8868,.T.);
#11625=ORIENTED_EDGE('',*,*,#8972,.T.);
#11626=ORIENTED_EDGE('',*,*,#8726,.F.);
#11627=ORIENTED_EDGE('',*,*,#8973,.F.);
#11628=ORIENTED_EDGE('',*,*,#8864,.T.);
#11629=ORIENTED_EDGE('',*,*,#8974,.T.);
#11630=ORIENTED_EDGE('',*,*,#8730,.F.);
#11631=ORIENTED_EDGE('',*,*,#8975,.F.);
#11632=ORIENTED_EDGE('',*,*,#8860,.T.);
#11633=ORIENTED_EDGE('',*,*,#8976,.T.);
#11634=ORIENTED_EDGE('',*,*,#8734,.F.);
#11635=ORIENTED_EDGE('',*,*,#8977,.F.);
#11636=ORIENTED_EDGE('',*,*,#8856,.T.);
#11637=ORIENTED_EDGE('',*,*,#8978,.T.);
#11638=ORIENTED_EDGE('',*,*,#8738,.F.);
#11639=ORIENTED_EDGE('',*,*,#8979,.F.);
#11640=ORIENTED_EDGE('',*,*,#8852,.T.);
#11641=ORIENTED_EDGE('',*,*,#8980,.T.);
#11642=ORIENTED_EDGE('',*,*,#8742,.F.);
#11643=ORIENTED_EDGE('',*,*,#8981,.F.);
#11644=ORIENTED_EDGE('',*,*,#8848,.T.);
#11645=ORIENTED_EDGE('',*,*,#8982,.T.);
#11646=ORIENTED_EDGE('',*,*,#8746,.F.);
#11647=ORIENTED_EDGE('',*,*,#8983,.F.);
#11648=ORIENTED_EDGE('',*,*,#8844,.T.);
#11649=ORIENTED_EDGE('',*,*,#8984,.T.);
#11650=ORIENTED_EDGE('',*,*,#8750,.F.);
#11651=ORIENTED_EDGE('',*,*,#8985,.F.);
#11652=ORIENTED_EDGE('',*,*,#8840,.T.);
#11653=ORIENTED_EDGE('',*,*,#8986,.T.);
#11654=ORIENTED_EDGE('',*,*,#8754,.F.);
#11655=ORIENTED_EDGE('',*,*,#8987,.F.);
#11656=ORIENTED_EDGE('',*,*,#8836,.T.);
#11657=ORIENTED_EDGE('',*,*,#8988,.T.);
#11658=ORIENTED_EDGE('',*,*,#8758,.F.);
#11659=ORIENTED_EDGE('',*,*,#8989,.F.);
#11660=ORIENTED_EDGE('',*,*,#8832,.T.);
#11661=ORIENTED_EDGE('',*,*,#8990,.T.);
#11662=ORIENTED_EDGE('',*,*,#8762,.F.);
#11663=ORIENTED_EDGE('',*,*,#8991,.F.);
#11664=ORIENTED_EDGE('',*,*,#8828,.T.);
#11665=ORIENTED_EDGE('',*,*,#8992,.T.);
#11666=ORIENTED_EDGE('',*,*,#8766,.F.);
#11667=ORIENTED_EDGE('',*,*,#8993,.F.);
#11668=ORIENTED_EDGE('',*,*,#8824,.T.);
#11669=ORIENTED_EDGE('',*,*,#8994,.T.);
#11670=ORIENTED_EDGE('',*,*,#8770,.F.);
#11671=ORIENTED_EDGE('',*,*,#8995,.F.);
#11672=ORIENTED_EDGE('',*,*,#8820,.T.);
#11673=ORIENTED_EDGE('',*,*,#8996,.T.);
#11674=ORIENTED_EDGE('',*,*,#8774,.F.);
#11675=ORIENTED_EDGE('',*,*,#8997,.F.);
#11676=ORIENTED_EDGE('',*,*,#8816,.T.);
#11677=ORIENTED_EDGE('',*,*,#8998,.T.);
#11678=ORIENTED_EDGE('',*,*,#8778,.F.);
#11679=ORIENTED_EDGE('',*,*,#8999,.F.);
#11680=ORIENTED_EDGE('',*,*,#8812,.T.);
#11681=ORIENTED_EDGE('',*,*,#9000,.T.);
#11682=ORIENTED_EDGE('',*,*,#8782,.F.);
#11683=ORIENTED_EDGE('',*,*,#9001,.F.);
#11684=ORIENTED_EDGE('',*,*,#8808,.T.);
#11685=ORIENTED_EDGE('',*,*,#9002,.T.);
#11686=ORIENTED_EDGE('',*,*,#8786,.F.);
#11687=ORIENTED_EDGE('',*,*,#9003,.F.);
#11688=ORIENTED_EDGE('',*,*,#8804,.T.);
#11689=ORIENTED_EDGE('',*,*,#9004,.T.);
#11690=ORIENTED_EDGE('',*,*,#9005,.F.);
#11691=ORIENTED_EDGE('',*,*,#8796,.T.);
#11692=ORIENTED_EDGE('',*,*,#9006,.T.);
#11693=ORIENTED_EDGE('',*,*,#8660,.F.);
#11694=ORIENTED_EDGE('',*,*,#8661,.T.);
#11695=ORIENTED_EDGE('',*,*,#9006,.F.);
#11696=ORIENTED_EDGE('',*,*,#8795,.F.);
#11697=ORIENTED_EDGE('',*,*,#9007,.T.);
#11698=ORIENTED_EDGE('',*,*,#8794,.F.);
#11699=ORIENTED_EDGE('',*,*,#9008,.T.);
#11700=ORIENTED_EDGE('',*,*,#8662,.T.);
#11701=ORIENTED_EDGE('',*,*,#9007,.F.);
#11702=ORIENTED_EDGE('',*,*,#8691,.T.);
#11703=ORIENTED_EDGE('',*,*,#8956,.F.);
#11704=ORIENTED_EDGE('',*,*,#8899,.F.);
#11705=ORIENTED_EDGE('',*,*,#9009,.T.);
#11706=ORIENTED_EDGE('',*,*,#8692,.T.);
#11707=ORIENTED_EDGE('',*,*,#9009,.F.);
#11708=ORIENTED_EDGE('',*,*,#8898,.F.);
#11709=ORIENTED_EDGE('',*,*,#9010,.T.);
#11710=ORIENTED_EDGE('',*,*,#8689,.F.);
#11711=ORIENTED_EDGE('',*,*,#9010,.F.);
#11712=ORIENTED_EDGE('',*,*,#8897,.T.);
#11713=ORIENTED_EDGE('',*,*,#8955,.T.);
#11714=ORIENTED_EDGE('',*,*,#8695,.T.);
#11715=ORIENTED_EDGE('',*,*,#8958,.F.);
#11716=ORIENTED_EDGE('',*,*,#8895,.F.);
#11717=ORIENTED_EDGE('',*,*,#9011,.T.);
#11718=ORIENTED_EDGE('',*,*,#8696,.T.);
#11719=ORIENTED_EDGE('',*,*,#9011,.F.);
#11720=ORIENTED_EDGE('',*,*,#8894,.F.);
#11721=ORIENTED_EDGE('',*,*,#9012,.T.);
#11722=ORIENTED_EDGE('',*,*,#8693,.F.);
#11723=ORIENTED_EDGE('',*,*,#9012,.F.);
#11724=ORIENTED_EDGE('',*,*,#8893,.T.);
#11725=ORIENTED_EDGE('',*,*,#8957,.T.);
#11726=ORIENTED_EDGE('',*,*,#8699,.T.);
#11727=ORIENTED_EDGE('',*,*,#8960,.F.);
#11728=ORIENTED_EDGE('',*,*,#8891,.F.);
#11729=ORIENTED_EDGE('',*,*,#9013,.T.);
#11730=ORIENTED_EDGE('',*,*,#8700,.T.);
#11731=ORIENTED_EDGE('',*,*,#9013,.F.);
#11732=ORIENTED_EDGE('',*,*,#8890,.F.);
#11733=ORIENTED_EDGE('',*,*,#9014,.T.);
#11734=ORIENTED_EDGE('',*,*,#8697,.F.);
#11735=ORIENTED_EDGE('',*,*,#9014,.F.);
#11736=ORIENTED_EDGE('',*,*,#8889,.T.);
#11737=ORIENTED_EDGE('',*,*,#8959,.T.);
#11738=ORIENTED_EDGE('',*,*,#8703,.T.);
#11739=ORIENTED_EDGE('',*,*,#8962,.F.);
#11740=ORIENTED_EDGE('',*,*,#8887,.F.);
#11741=ORIENTED_EDGE('',*,*,#9015,.T.);
#11742=ORIENTED_EDGE('',*,*,#8704,.T.);
#11743=ORIENTED_EDGE('',*,*,#9015,.F.);
#11744=ORIENTED_EDGE('',*,*,#8886,.F.);
#11745=ORIENTED_EDGE('',*,*,#9016,.T.);
#11746=ORIENTED_EDGE('',*,*,#8701,.F.);
#11747=ORIENTED_EDGE('',*,*,#9016,.F.);
#11748=ORIENTED_EDGE('',*,*,#8885,.T.);
#11749=ORIENTED_EDGE('',*,*,#8961,.T.);
#11750=ORIENTED_EDGE('',*,*,#8707,.T.);
#11751=ORIENTED_EDGE('',*,*,#8964,.F.);
#11752=ORIENTED_EDGE('',*,*,#8883,.F.);
#11753=ORIENTED_EDGE('',*,*,#9017,.T.);
#11754=ORIENTED_EDGE('',*,*,#8708,.T.);
#11755=ORIENTED_EDGE('',*,*,#9017,.F.);
#11756=ORIENTED_EDGE('',*,*,#8882,.F.);
#11757=ORIENTED_EDGE('',*,*,#9018,.T.);
#11758=ORIENTED_EDGE('',*,*,#8705,.F.);
#11759=ORIENTED_EDGE('',*,*,#9018,.F.);
#11760=ORIENTED_EDGE('',*,*,#8881,.T.);
#11761=ORIENTED_EDGE('',*,*,#8963,.T.);
#11762=ORIENTED_EDGE('',*,*,#8711,.T.);
#11763=ORIENTED_EDGE('',*,*,#8966,.F.);
#11764=ORIENTED_EDGE('',*,*,#8879,.F.);
#11765=ORIENTED_EDGE('',*,*,#9019,.T.);
#11766=ORIENTED_EDGE('',*,*,#8712,.T.);
#11767=ORIENTED_EDGE('',*,*,#9019,.F.);
#11768=ORIENTED_EDGE('',*,*,#8878,.F.);
#11769=ORIENTED_EDGE('',*,*,#9020,.T.);
#11770=ORIENTED_EDGE('',*,*,#8709,.F.);
#11771=ORIENTED_EDGE('',*,*,#9020,.F.);
#11772=ORIENTED_EDGE('',*,*,#8877,.T.);
#11773=ORIENTED_EDGE('',*,*,#8965,.T.);
#11774=ORIENTED_EDGE('',*,*,#8715,.T.);
#11775=ORIENTED_EDGE('',*,*,#8968,.F.);
#11776=ORIENTED_EDGE('',*,*,#8875,.F.);
#11777=ORIENTED_EDGE('',*,*,#9021,.T.);
#11778=ORIENTED_EDGE('',*,*,#8716,.T.);
#11779=ORIENTED_EDGE('',*,*,#9021,.F.);
#11780=ORIENTED_EDGE('',*,*,#8874,.F.);
#11781=ORIENTED_EDGE('',*,*,#9022,.T.);
#11782=ORIENTED_EDGE('',*,*,#8713,.F.);
#11783=ORIENTED_EDGE('',*,*,#9022,.F.);
#11784=ORIENTED_EDGE('',*,*,#8873,.T.);
#11785=ORIENTED_EDGE('',*,*,#8967,.T.);
#11786=ORIENTED_EDGE('',*,*,#8719,.T.);
#11787=ORIENTED_EDGE('',*,*,#8970,.F.);
#11788=ORIENTED_EDGE('',*,*,#8871,.F.);
#11789=ORIENTED_EDGE('',*,*,#9023,.T.);
#11790=ORIENTED_EDGE('',*,*,#8720,.T.);
#11791=ORIENTED_EDGE('',*,*,#9023,.F.);
#11792=ORIENTED_EDGE('',*,*,#8870,.F.);
#11793=ORIENTED_EDGE('',*,*,#9024,.T.);
#11794=ORIENTED_EDGE('',*,*,#8717,.F.);
#11795=ORIENTED_EDGE('',*,*,#9024,.F.);
#11796=ORIENTED_EDGE('',*,*,#8869,.T.);
#11797=ORIENTED_EDGE('',*,*,#8969,.T.);
#11798=ORIENTED_EDGE('',*,*,#8723,.T.);
#11799=ORIENTED_EDGE('',*,*,#8972,.F.);
#11800=ORIENTED_EDGE('',*,*,#8867,.F.);
#11801=ORIENTED_EDGE('',*,*,#9025,.T.);
#11802=ORIENTED_EDGE('',*,*,#8724,.T.);
#11803=ORIENTED_EDGE('',*,*,#9025,.F.);
#11804=ORIENTED_EDGE('',*,*,#8866,.F.);
#11805=ORIENTED_EDGE('',*,*,#9026,.T.);
#11806=ORIENTED_EDGE('',*,*,#8721,.F.);
#11807=ORIENTED_EDGE('',*,*,#9026,.F.);
#11808=ORIENTED_EDGE('',*,*,#8865,.T.);
#11809=ORIENTED_EDGE('',*,*,#8971,.T.);
#11810=ORIENTED_EDGE('',*,*,#8727,.T.);
#11811=ORIENTED_EDGE('',*,*,#8974,.F.);
#11812=ORIENTED_EDGE('',*,*,#8863,.F.);
#11813=ORIENTED_EDGE('',*,*,#9027,.T.);
#11814=ORIENTED_EDGE('',*,*,#8728,.T.);
#11815=ORIENTED_EDGE('',*,*,#9027,.F.);
#11816=ORIENTED_EDGE('',*,*,#8862,.F.);
#11817=ORIENTED_EDGE('',*,*,#9028,.T.);
#11818=ORIENTED_EDGE('',*,*,#8725,.F.);
#11819=ORIENTED_EDGE('',*,*,#9028,.F.);
#11820=ORIENTED_EDGE('',*,*,#8861,.T.);
#11821=ORIENTED_EDGE('',*,*,#8973,.T.);
#11822=ORIENTED_EDGE('',*,*,#8731,.T.);
#11823=ORIENTED_EDGE('',*,*,#8976,.F.);
#11824=ORIENTED_EDGE('',*,*,#8859,.F.);
#11825=ORIENTED_EDGE('',*,*,#9029,.T.);
#11826=ORIENTED_EDGE('',*,*,#8732,.T.);
#11827=ORIENTED_EDGE('',*,*,#9029,.F.);
#11828=ORIENTED_EDGE('',*,*,#8858,.F.);
#11829=ORIENTED_EDGE('',*,*,#9030,.T.);
#11830=ORIENTED_EDGE('',*,*,#8729,.F.);
#11831=ORIENTED_EDGE('',*,*,#9030,.F.);
#11832=ORIENTED_EDGE('',*,*,#8857,.T.);
#11833=ORIENTED_EDGE('',*,*,#8975,.T.);
#11834=ORIENTED_EDGE('',*,*,#8735,.T.);
#11835=ORIENTED_EDGE('',*,*,#8978,.F.);
#11836=ORIENTED_EDGE('',*,*,#8855,.F.);
#11837=ORIENTED_EDGE('',*,*,#9031,.T.);
#11838=ORIENTED_EDGE('',*,*,#8736,.T.);
#11839=ORIENTED_EDGE('',*,*,#9031,.F.);
#11840=ORIENTED_EDGE('',*,*,#8854,.F.);
#11841=ORIENTED_EDGE('',*,*,#9032,.T.);
#11842=ORIENTED_EDGE('',*,*,#8733,.F.);
#11843=ORIENTED_EDGE('',*,*,#9032,.F.);
#11844=ORIENTED_EDGE('',*,*,#8853,.T.);
#11845=ORIENTED_EDGE('',*,*,#8977,.T.);
#11846=ORIENTED_EDGE('',*,*,#8739,.T.);
#11847=ORIENTED_EDGE('',*,*,#8980,.F.);
#11848=ORIENTED_EDGE('',*,*,#8851,.F.);
#11849=ORIENTED_EDGE('',*,*,#9033,.T.);
#11850=ORIENTED_EDGE('',*,*,#8740,.T.);
#11851=ORIENTED_EDGE('',*,*,#9033,.F.);
#11852=ORIENTED_EDGE('',*,*,#8850,.F.);
#11853=ORIENTED_EDGE('',*,*,#9034,.T.);
#11854=ORIENTED_EDGE('',*,*,#8737,.F.);
#11855=ORIENTED_EDGE('',*,*,#9034,.F.);
#11856=ORIENTED_EDGE('',*,*,#8849,.T.);
#11857=ORIENTED_EDGE('',*,*,#8979,.T.);
#11858=ORIENTED_EDGE('',*,*,#8743,.T.);
#11859=ORIENTED_EDGE('',*,*,#8982,.F.);
#11860=ORIENTED_EDGE('',*,*,#8847,.F.);
#11861=ORIENTED_EDGE('',*,*,#9035,.T.);
#11862=ORIENTED_EDGE('',*,*,#8744,.T.);
#11863=ORIENTED_EDGE('',*,*,#9035,.F.);
#11864=ORIENTED_EDGE('',*,*,#8846,.F.);
#11865=ORIENTED_EDGE('',*,*,#9036,.T.);
#11866=ORIENTED_EDGE('',*,*,#8741,.F.);
#11867=ORIENTED_EDGE('',*,*,#9036,.F.);
#11868=ORIENTED_EDGE('',*,*,#8845,.T.);
#11869=ORIENTED_EDGE('',*,*,#8981,.T.);
#11870=ORIENTED_EDGE('',*,*,#8747,.T.);
#11871=ORIENTED_EDGE('',*,*,#8984,.F.);
#11872=ORIENTED_EDGE('',*,*,#8843,.F.);
#11873=ORIENTED_EDGE('',*,*,#9037,.T.);
#11874=ORIENTED_EDGE('',*,*,#8748,.T.);
#11875=ORIENTED_EDGE('',*,*,#9037,.F.);
#11876=ORIENTED_EDGE('',*,*,#8842,.F.);
#11877=ORIENTED_EDGE('',*,*,#9038,.T.);
#11878=ORIENTED_EDGE('',*,*,#8745,.F.);
#11879=ORIENTED_EDGE('',*,*,#9038,.F.);
#11880=ORIENTED_EDGE('',*,*,#8841,.T.);
#11881=ORIENTED_EDGE('',*,*,#8983,.T.);
#11882=ORIENTED_EDGE('',*,*,#8751,.T.);
#11883=ORIENTED_EDGE('',*,*,#8986,.F.);
#11884=ORIENTED_EDGE('',*,*,#8839,.F.);
#11885=ORIENTED_EDGE('',*,*,#9039,.T.);
#11886=ORIENTED_EDGE('',*,*,#8752,.T.);
#11887=ORIENTED_EDGE('',*,*,#9039,.F.);
#11888=ORIENTED_EDGE('',*,*,#8838,.F.);
#11889=ORIENTED_EDGE('',*,*,#9040,.T.);
#11890=ORIENTED_EDGE('',*,*,#8749,.F.);
#11891=ORIENTED_EDGE('',*,*,#9040,.F.);
#11892=ORIENTED_EDGE('',*,*,#8837,.T.);
#11893=ORIENTED_EDGE('',*,*,#8985,.T.);
#11894=ORIENTED_EDGE('',*,*,#8755,.T.);
#11895=ORIENTED_EDGE('',*,*,#8988,.F.);
#11896=ORIENTED_EDGE('',*,*,#8835,.F.);
#11897=ORIENTED_EDGE('',*,*,#9041,.T.);
#11898=ORIENTED_EDGE('',*,*,#8756,.T.);
#11899=ORIENTED_EDGE('',*,*,#9041,.F.);
#11900=ORIENTED_EDGE('',*,*,#8834,.F.);
#11901=ORIENTED_EDGE('',*,*,#9042,.T.);
#11902=ORIENTED_EDGE('',*,*,#8753,.F.);
#11903=ORIENTED_EDGE('',*,*,#9042,.F.);
#11904=ORIENTED_EDGE('',*,*,#8833,.T.);
#11905=ORIENTED_EDGE('',*,*,#8987,.T.);
#11906=ORIENTED_EDGE('',*,*,#8759,.T.);
#11907=ORIENTED_EDGE('',*,*,#8990,.F.);
#11908=ORIENTED_EDGE('',*,*,#8831,.F.);
#11909=ORIENTED_EDGE('',*,*,#9043,.T.);
#11910=ORIENTED_EDGE('',*,*,#8760,.T.);
#11911=ORIENTED_EDGE('',*,*,#9043,.F.);
#11912=ORIENTED_EDGE('',*,*,#8830,.F.);
#11913=ORIENTED_EDGE('',*,*,#9044,.T.);
#11914=ORIENTED_EDGE('',*,*,#8757,.F.);
#11915=ORIENTED_EDGE('',*,*,#9044,.F.);
#11916=ORIENTED_EDGE('',*,*,#8829,.T.);
#11917=ORIENTED_EDGE('',*,*,#8989,.T.);
#11918=ORIENTED_EDGE('',*,*,#8763,.T.);
#11919=ORIENTED_EDGE('',*,*,#8992,.F.);
#11920=ORIENTED_EDGE('',*,*,#8827,.F.);
#11921=ORIENTED_EDGE('',*,*,#9045,.T.);
#11922=ORIENTED_EDGE('',*,*,#8764,.T.);
#11923=ORIENTED_EDGE('',*,*,#9045,.F.);
#11924=ORIENTED_EDGE('',*,*,#8826,.F.);
#11925=ORIENTED_EDGE('',*,*,#9046,.T.);
#11926=ORIENTED_EDGE('',*,*,#8761,.F.);
#11927=ORIENTED_EDGE('',*,*,#9046,.F.);
#11928=ORIENTED_EDGE('',*,*,#8825,.T.);
#11929=ORIENTED_EDGE('',*,*,#8991,.T.);
#11930=ORIENTED_EDGE('',*,*,#8767,.T.);
#11931=ORIENTED_EDGE('',*,*,#8994,.F.);
#11932=ORIENTED_EDGE('',*,*,#8823,.F.);
#11933=ORIENTED_EDGE('',*,*,#9047,.T.);
#11934=ORIENTED_EDGE('',*,*,#8768,.T.);
#11935=ORIENTED_EDGE('',*,*,#9047,.F.);
#11936=ORIENTED_EDGE('',*,*,#8822,.F.);
#11937=ORIENTED_EDGE('',*,*,#9048,.T.);
#11938=ORIENTED_EDGE('',*,*,#8765,.F.);
#11939=ORIENTED_EDGE('',*,*,#9048,.F.);
#11940=ORIENTED_EDGE('',*,*,#8821,.T.);
#11941=ORIENTED_EDGE('',*,*,#8993,.T.);
#11942=ORIENTED_EDGE('',*,*,#8771,.T.);
#11943=ORIENTED_EDGE('',*,*,#8996,.F.);
#11944=ORIENTED_EDGE('',*,*,#8819,.F.);
#11945=ORIENTED_EDGE('',*,*,#9049,.T.);
#11946=ORIENTED_EDGE('',*,*,#8772,.T.);
#11947=ORIENTED_EDGE('',*,*,#9049,.F.);
#11948=ORIENTED_EDGE('',*,*,#8818,.F.);
#11949=ORIENTED_EDGE('',*,*,#9050,.T.);
#11950=ORIENTED_EDGE('',*,*,#8769,.F.);
#11951=ORIENTED_EDGE('',*,*,#9050,.F.);
#11952=ORIENTED_EDGE('',*,*,#8817,.T.);
#11953=ORIENTED_EDGE('',*,*,#8995,.T.);
#11954=ORIENTED_EDGE('',*,*,#8775,.T.);
#11955=ORIENTED_EDGE('',*,*,#8998,.F.);
#11956=ORIENTED_EDGE('',*,*,#8815,.F.);
#11957=ORIENTED_EDGE('',*,*,#9051,.T.);
#11958=ORIENTED_EDGE('',*,*,#8776,.T.);
#11959=ORIENTED_EDGE('',*,*,#9051,.F.);
#11960=ORIENTED_EDGE('',*,*,#8814,.F.);
#11961=ORIENTED_EDGE('',*,*,#9052,.T.);
#11962=ORIENTED_EDGE('',*,*,#8773,.F.);
#11963=ORIENTED_EDGE('',*,*,#9052,.F.);
#11964=ORIENTED_EDGE('',*,*,#8813,.T.);
#11965=ORIENTED_EDGE('',*,*,#8997,.T.);
#11966=ORIENTED_EDGE('',*,*,#8779,.T.);
#11967=ORIENTED_EDGE('',*,*,#9000,.F.);
#11968=ORIENTED_EDGE('',*,*,#8811,.F.);
#11969=ORIENTED_EDGE('',*,*,#9053,.T.);
#11970=ORIENTED_EDGE('',*,*,#8780,.T.);
#11971=ORIENTED_EDGE('',*,*,#9053,.F.);
#11972=ORIENTED_EDGE('',*,*,#8810,.F.);
#11973=ORIENTED_EDGE('',*,*,#9054,.T.);
#11974=ORIENTED_EDGE('',*,*,#8777,.F.);
#11975=ORIENTED_EDGE('',*,*,#9054,.F.);
#11976=ORIENTED_EDGE('',*,*,#8809,.T.);
#11977=ORIENTED_EDGE('',*,*,#8999,.T.);
#11978=ORIENTED_EDGE('',*,*,#8783,.T.);
#11979=ORIENTED_EDGE('',*,*,#9002,.F.);
#11980=ORIENTED_EDGE('',*,*,#8807,.F.);
#11981=ORIENTED_EDGE('',*,*,#9055,.T.);
#11982=ORIENTED_EDGE('',*,*,#8784,.T.);
#11983=ORIENTED_EDGE('',*,*,#9055,.F.);
#11984=ORIENTED_EDGE('',*,*,#8806,.F.);
#11985=ORIENTED_EDGE('',*,*,#9056,.T.);
#11986=ORIENTED_EDGE('',*,*,#8781,.F.);
#11987=ORIENTED_EDGE('',*,*,#9056,.F.);
#11988=ORIENTED_EDGE('',*,*,#8805,.T.);
#11989=ORIENTED_EDGE('',*,*,#9001,.T.);
#11990=ORIENTED_EDGE('',*,*,#8787,.T.);
#11991=ORIENTED_EDGE('',*,*,#9004,.F.);
#11992=ORIENTED_EDGE('',*,*,#8803,.F.);
#11993=ORIENTED_EDGE('',*,*,#9057,.T.);
#11994=ORIENTED_EDGE('',*,*,#8788,.T.);
#11995=ORIENTED_EDGE('',*,*,#9057,.F.);
#11996=ORIENTED_EDGE('',*,*,#8802,.F.);
#11997=ORIENTED_EDGE('',*,*,#9058,.T.);
#11998=ORIENTED_EDGE('',*,*,#8785,.F.);
#11999=ORIENTED_EDGE('',*,*,#9058,.F.);
#12000=ORIENTED_EDGE('',*,*,#8801,.T.);
#12001=ORIENTED_EDGE('',*,*,#9003,.T.);
#12002=ORIENTED_EDGE('',*,*,#8791,.T.);
#12003=ORIENTED_EDGE('',*,*,#8928,.F.);
#12004=ORIENTED_EDGE('',*,*,#8799,.F.);
#12005=ORIENTED_EDGE('',*,*,#9059,.T.);
#12006=ORIENTED_EDGE('',*,*,#8792,.T.);
#12007=ORIENTED_EDGE('',*,*,#9059,.F.);
#12008=ORIENTED_EDGE('',*,*,#8798,.F.);
#12009=ORIENTED_EDGE('',*,*,#9060,.T.);
#12010=ORIENTED_EDGE('',*,*,#8789,.F.);
#12011=ORIENTED_EDGE('',*,*,#9060,.F.);
#12012=ORIENTED_EDGE('',*,*,#8797,.T.);
#12013=ORIENTED_EDGE('',*,*,#8927,.T.);
#12014=ORIENTED_EDGE('',*,*,#9005,.T.);
#12015=ORIENTED_EDGE('',*,*,#8659,.T.);
#12016=ORIENTED_EDGE('',*,*,#9008,.F.);
#12017=ORIENTED_EDGE('',*,*,#8793,.T.);
#16324=PLANE('',#17917);
#16325=PLANE('',#17944);
#16326=PLANE('',#17971);
#16327=PLANE('',#17998);
#16328=PLANE('',#17999);
#16329=PLANE('',#18000);
#16330=PLANE('',#18001);
#16331=PLANE('',#18002);
#16332=PLANE('',#18003);
#16333=PLANE('',#18004);
#16334=PLANE('',#18005);
#16335=PLANE('',#18006);
#16336=PLANE('',#18007);
#16337=PLANE('',#18008);
#16338=PLANE('',#18009);
#16339=PLANE('',#18010);
#16340=PLANE('',#18011);
#16341=PLANE('',#18012);
#16342=PLANE('',#18013);
#16343=PLANE('',#18014);
#16344=PLANE('',#18015);
#16345=PLANE('',#18016);
#16346=PLANE('',#18017);
#16347=PLANE('',#18018);
#16348=PLANE('',#18019);
#16349=PLANE('',#18020);
#16350=PLANE('',#18021);
#16351=PLANE('',#18022);
#16352=PLANE('',#18023);
#16353=PLANE('',#18024);
#16354=PLANE('',#18025);
#16355=PLANE('',#18026);
#16356=PLANE('',#18027);
#16357=PLANE('',#18028);
#16358=PLANE('',#18029);
#16359=PLANE('',#18030);
#16360=PLANE('',#18031);
#16361=PLANE('',#18032);
#16362=PLANE('',#18033);
#16363=PLANE('',#18034);
#16364=PLANE('',#18035);
#16365=PLANE('',#18036);
#16366=PLANE('',#18037);
#16367=PLANE('',#18038);
#16368=PLANE('',#18039);
#16369=PLANE('',#18040);
#16370=PLANE('',#18041);
#16371=PLANE('',#18042);
#16372=PLANE('',#18043);
#16373=PLANE('',#18044);
#16374=PLANE('',#18045);
#16375=PLANE('',#18046);
#16376=PLANE('',#18047);
#16377=PLANE('',#18048);
#16378=PLANE('',#18049);
#16379=PLANE('',#18050);
#16380=PLANE('',#18051);
#16381=PLANE('',#18052);
#16382=PLANE('',#18053);
#16383=PLANE('',#18054);
#16384=PLANE('',#18055);
#16385=PLANE('',#18056);
#16386=PLANE('',#18057);
#16387=PLANE('',#18058);
#16388=PLANE('',#18059);
#16389=PLANE('',#18060);
#16390=PLANE('',#18061);
#16391=PLANE('',#18062);
#16392=PLANE('',#18063);
#16393=PLANE('',#18064);
#16394=PLANE('',#18065);
#16395=PLANE('',#18066);
#16396=PLANE('',#18067);
#16397=PLANE('',#18068);
#16398=PLANE('',#18069);
#16399=PLANE('',#18070);
#16400=PLANE('',#18071);
#16401=PLANE('',#18072);
#16402=PLANE('',#18073);
#16403=PLANE('',#18074);
#16404=PLANE('',#18075);
#16405=PLANE('',#18076);
#16406=PLANE('',#18077);
#16407=PLANE('',#18078);
#16408=PLANE('',#18079);
#16409=PLANE('',#18080);
#16410=PLANE('',#18081);
#16411=PLANE('',#18082);
#16412=PLANE('',#18083);
#16413=PLANE('',#18084);
#16414=PLANE('',#18085);
#16415=PLANE('',#18086);
#16416=PLANE('',#18087);
#16417=PLANE('',#18088);
#16418=PLANE('',#18089);
#16419=PLANE('',#18090);
#16420=PLANE('',#18091);
#16421=PLANE('',#18092);
#16422=PLANE('',#18093);
#16423=PLANE('',#18094);
#16424=PLANE('',#18095);
#16425=PLANE('',#18096);
#16426=PLANE('',#18097);
#16427=PLANE('',#18098);
#16428=PLANE('',#18099);
#16429=PLANE('',#18100);
#16430=PLANE('',#18101);
#16431=PLANE('',#18102);
#16432=PLANE('',#18103);
#16433=PLANE('',#18104);
#16862=ADVANCED_FACE('',(#1527,#776,#777,#778,#779,#780,#781,#782,#783,
#784,#785,#786,#787,#788,#789,#790,#791,#792,#793,#794,#795,#796,#797,#798,
#799,#800,#801,#802,#803,#804,#805,#806,#807,#808,#809,#810,#811,#812,#813,
#814,#815,#816,#817,#818,#819,#820,#821,#822,#823,#824,#825,#826,#827),
#16324,.F.);
#16863=ADVANCED_FACE('',(#1528,#828,#829,#830,#831,#832,#833,#834,#835,
#836,#837,#838,#839,#840,#841,#842,#843,#844,#845,#846,#847,#848,#849,#850,
#851,#852,#853,#854,#855,#856,#857,#858,#859,#860,#861,#862,#863,#864,#865,
#866,#867,#868,#869,#870,#871,#872,#873,#874,#875,#876,#877,#878,#879),
#16325,.T.);
#16864=ADVANCED_FACE('',(#1529),#16326,.T.);
#16865=ADVANCED_FACE('',(#1530),#489,.F.);
#16866=ADVANCED_FACE('',(#1531),#490,.F.);
#16867=ADVANCED_FACE('',(#1532),#491,.F.);
#16868=ADVANCED_FACE('',(#1533),#492,.F.);
#16869=ADVANCED_FACE('',(#1534),#493,.F.);
#16870=ADVANCED_FACE('',(#1535),#494,.F.);
#16871=ADVANCED_FACE('',(#1536),#495,.F.);
#16872=ADVANCED_FACE('',(#1537),#496,.F.);
#16873=ADVANCED_FACE('',(#1538),#497,.F.);
#16874=ADVANCED_FACE('',(#1539),#498,.F.);
#16875=ADVANCED_FACE('',(#1540),#499,.F.);
#16876=ADVANCED_FACE('',(#1541),#500,.F.);
#16877=ADVANCED_FACE('',(#1542),#501,.F.);
#16878=ADVANCED_FACE('',(#1543),#502,.F.);
#16879=ADVANCED_FACE('',(#1544),#503,.F.);
#16880=ADVANCED_FACE('',(#1545),#504,.F.);
#16881=ADVANCED_FACE('',(#1546),#505,.F.);
#16882=ADVANCED_FACE('',(#1547),#506,.F.);
#16883=ADVANCED_FACE('',(#1548),#507,.F.);
#16884=ADVANCED_FACE('',(#1549),#508,.F.);
#16885=ADVANCED_FACE('',(#1550),#509,.F.);
#16886=ADVANCED_FACE('',(#1551),#510,.F.);
#16887=ADVANCED_FACE('',(#1552),#511,.F.);
#16888=ADVANCED_FACE('',(#1553),#512,.F.);
#16889=ADVANCED_FACE('',(#1554),#513,.F.);
#16890=ADVANCED_FACE('',(#1555),#514,.F.);
#16891=ADVANCED_FACE('',(#1556),#16327,.T.);
#16892=ADVANCED_FACE('',(#1557),#16328,.T.);
#16893=ADVANCED_FACE('',(#1558),#16329,.T.);
#16894=ADVANCED_FACE('',(#1559),#16330,.T.);
#16895=ADVANCED_FACE('',(#1560),#16331,.T.);
#16896=ADVANCED_FACE('',(#1561),#16332,.T.);
#16897=ADVANCED_FACE('',(#1562),#16333,.T.);
#16898=ADVANCED_FACE('',(#1563),#16334,.T.);
#16899=ADVANCED_FACE('',(#1564),#16335,.T.);
#16900=ADVANCED_FACE('',(#1565),#16336,.T.);
#16901=ADVANCED_FACE('',(#1566),#16337,.T.);
#16902=ADVANCED_FACE('',(#1567),#16338,.T.);
#16903=ADVANCED_FACE('',(#1568),#16339,.T.);
#16904=ADVANCED_FACE('',(#1569),#16340,.T.);
#16905=ADVANCED_FACE('',(#1570),#16341,.T.);
#16906=ADVANCED_FACE('',(#1571),#16342,.T.);
#16907=ADVANCED_FACE('',(#1572),#16343,.T.);
#16908=ADVANCED_FACE('',(#1573),#16344,.T.);
#16909=ADVANCED_FACE('',(#1574),#16345,.T.);
#16910=ADVANCED_FACE('',(#1575),#16346,.T.);
#16911=ADVANCED_FACE('',(#1576),#16347,.T.);
#16912=ADVANCED_FACE('',(#1577),#16348,.T.);
#16913=ADVANCED_FACE('',(#1578),#16349,.T.);
#16914=ADVANCED_FACE('',(#1579),#16350,.T.);
#16915=ADVANCED_FACE('',(#1580),#16351,.T.);
#16916=ADVANCED_FACE('',(#1581),#16352,.T.);
#16917=ADVANCED_FACE('',(#1582),#16353,.F.);
#16918=ADVANCED_FACE('',(#1583),#16354,.F.);
#16919=ADVANCED_FACE('',(#1584),#16355,.F.);
#16920=ADVANCED_FACE('',(#1585),#16356,.F.);
#16921=ADVANCED_FACE('',(#1586),#16357,.T.);
#16922=ADVANCED_FACE('',(#1587),#16358,.F.);
#16923=ADVANCED_FACE('',(#1588),#16359,.F.);
#16924=ADVANCED_FACE('',(#1589),#16360,.T.);
#16925=ADVANCED_FACE('',(#1590),#16361,.F.);
#16926=ADVANCED_FACE('',(#1591),#16362,.F.);
#16927=ADVANCED_FACE('',(#1592),#16363,.T.);
#16928=ADVANCED_FACE('',(#1593),#16364,.F.);
#16929=ADVANCED_FACE('',(#1594),#16365,.F.);
#16930=ADVANCED_FACE('',(#1595),#16366,.T.);
#16931=ADVANCED_FACE('',(#1596),#16367,.F.);
#16932=ADVANCED_FACE('',(#1597),#16368,.F.);
#16933=ADVANCED_FACE('',(#1598),#16369,.T.);
#16934=ADVANCED_FACE('',(#1599),#16370,.F.);
#16935=ADVANCED_FACE('',(#1600),#16371,.F.);
#16936=ADVANCED_FACE('',(#1601),#16372,.T.);
#16937=ADVANCED_FACE('',(#1602),#16373,.F.);
#16938=ADVANCED_FACE('',(#1603),#16374,.F.);
#16939=ADVANCED_FACE('',(#1604),#16375,.T.);
#16940=ADVANCED_FACE('',(#1605),#16376,.F.);
#16941=ADVANCED_FACE('',(#1606),#16377,.F.);
#16942=ADVANCED_FACE('',(#1607),#16378,.T.);
#16943=ADVANCED_FACE('',(#1608),#16379,.F.);
#16944=ADVANCED_FACE('',(#1609),#16380,.F.);
#16945=ADVANCED_FACE('',(#1610),#16381,.T.);
#16946=ADVANCED_FACE('',(#1611),#16382,.F.);
#16947=ADVANCED_FACE('',(#1612),#16383,.F.);
#16948=ADVANCED_FACE('',(#1613),#16384,.T.);
#16949=ADVANCED_FACE('',(#1614),#16385,.F.);
#16950=ADVANCED_FACE('',(#1615),#16386,.F.);
#16951=ADVANCED_FACE('',(#1616),#16387,.T.);
#16952=ADVANCED_FACE('',(#1617),#16388,.F.);
#16953=ADVANCED_FACE('',(#1618),#16389,.F.);
#16954=ADVANCED_FACE('',(#1619),#16390,.T.);
#16955=ADVANCED_FACE('',(#1620),#16391,.F.);
#16956=ADVANCED_FACE('',(#1621),#16392,.F.);
#16957=ADVANCED_FACE('',(#1622),#16393,.T.);
#16958=ADVANCED_FACE('',(#1623),#16394,.F.);
#16959=ADVANCED_FACE('',(#1624),#16395,.F.);
#16960=ADVANCED_FACE('',(#1625),#16396,.T.);
#16961=ADVANCED_FACE('',(#1626),#16397,.F.);
#16962=ADVANCED_FACE('',(#1627),#16398,.F.);
#16963=ADVANCED_FACE('',(#1628),#16399,.T.);
#16964=ADVANCED_FACE('',(#1629),#16400,.F.);
#16965=ADVANCED_FACE('',(#1630),#16401,.F.);
#16966=ADVANCED_FACE('',(#1631),#16402,.T.);
#16967=ADVANCED_FACE('',(#1632),#16403,.F.);
#16968=ADVANCED_FACE('',(#1633),#16404,.F.);
#16969=ADVANCED_FACE('',(#1634),#16405,.T.);
#16970=ADVANCED_FACE('',(#1635),#16406,.F.);
#16971=ADVANCED_FACE('',(#1636),#16407,.F.);
#16972=ADVANCED_FACE('',(#1637),#16408,.T.);
#16973=ADVANCED_FACE('',(#1638),#16409,.F.);
#16974=ADVANCED_FACE('',(#1639),#16410,.F.);
#16975=ADVANCED_FACE('',(#1640),#16411,.T.);
#16976=ADVANCED_FACE('',(#1641),#16412,.F.);
#16977=ADVANCED_FACE('',(#1642),#16413,.F.);
#16978=ADVANCED_FACE('',(#1643),#16414,.T.);
#16979=ADVANCED_FACE('',(#1644),#16415,.F.);
#16980=ADVANCED_FACE('',(#1645),#16416,.F.);
#16981=ADVANCED_FACE('',(#1646),#16417,.T.);
#16982=ADVANCED_FACE('',(#1647),#16418,.F.);
#16983=ADVANCED_FACE('',(#1648),#16419,.F.);
#16984=ADVANCED_FACE('',(#1649),#16420,.T.);
#16985=ADVANCED_FACE('',(#1650),#16421,.F.);
#16986=ADVANCED_FACE('',(#1651),#16422,.F.);
#16987=ADVANCED_FACE('',(#1652),#16423,.T.);
#16988=ADVANCED_FACE('',(#1653),#16424,.F.);
#16989=ADVANCED_FACE('',(#1654),#16425,.F.);
#16990=ADVANCED_FACE('',(#1655),#16426,.T.);
#16991=ADVANCED_FACE('',(#1656),#16427,.F.);
#16992=ADVANCED_FACE('',(#1657),#16428,.F.);
#16993=ADVANCED_FACE('',(#1658),#16429,.T.);
#16994=ADVANCED_FACE('',(#1659),#16430,.F.);
#16995=ADVANCED_FACE('',(#1660),#16431,.F.);
#16996=ADVANCED_FACE('',(#1661),#16432,.T.);
#16997=ADVANCED_FACE('',(#1662),#16433,.F.);
#17793=CLOSED_SHELL('',(#16862,#16863,#16864,#16865,#16866,#16867,#16868,
#16869,#16870,#16871,#16872,#16873,#16874,#16875,#16876,#16877,#16878,#16879,
#16880,#16881,#16882,#16883,#16884,#16885,#16886,#16887,#16888,#16889,#16890,
#16891,#16892,#16893,#16894,#16895,#16896,#16897,#16898,#16899,#16900,#16901,
#16902,#16903,#16904,#16905,#16906,#16907,#16908,#16909,#16910,#16911,#16912,
#16913,#16914,#16915,#16916,#16917,#16918,#16919,#16920,#16921,#16922,#16923,
#16924,#16925,#16926,#16927,#16928,#16929,#16930,#16931,#16932,#16933,#16934,
#16935,#16936,#16937,#16938,#16939,#16940,#16941,#16942,#16943,#16944,#16945,
#16946,#16947,#16948,#16949,#16950,#16951,#16952,#16953,#16954,#16955,#16956,
#16957,#16958,#16959,#16960,#16961,#16962,#16963,#16964,#16965,#16966,#16967,
#16968,#16969,#16970,#16971,#16972,#16973,#16974,#16975,#16976,#16977,#16978,
#16979,#16980,#16981,#16982,#16983,#16984,#16985,#16986,#16987,#16988,#16989,
#16990,#16991,#16992,#16993,#16994,#16995,#16996,#16997));
#17916=AXIS2_PLACEMENT_3D('',#24195,#19440,#19441);
#17917=AXIS2_PLACEMENT_3D('',#24196,#19442,#19443);
#17918=AXIS2_PLACEMENT_3D('',#24206,#19448,#19449);
#17919=AXIS2_PLACEMENT_3D('',#24208,#19450,#19451);
#17920=AXIS2_PLACEMENT_3D('',#24210,#19452,#19453);
#17921=AXIS2_PLACEMENT_3D('',#24212,#19454,#19455);
#17922=AXIS2_PLACEMENT_3D('',#24214,#19456,#19457);
#17923=AXIS2_PLACEMENT_3D('',#24216,#19458,#19459);
#17924=AXIS2_PLACEMENT_3D('',#24218,#19460,#19461);
#17925=AXIS2_PLACEMENT_3D('',#24220,#19462,#19463);
#17926=AXIS2_PLACEMENT_3D('',#24222,#19464,#19465);
#17927=AXIS2_PLACEMENT_3D('',#24224,#19466,#19467);
#17928=AXIS2_PLACEMENT_3D('',#24226,#19468,#19469);
#17929=AXIS2_PLACEMENT_3D('',#24228,#19470,#19471);
#17930=AXIS2_PLACEMENT_3D('',#24230,#19472,#19473);
#17931=AXIS2_PLACEMENT_3D('',#24232,#19474,#19475);
#17932=AXIS2_PLACEMENT_3D('',#24234,#19476,#19477);
#17933=AXIS2_PLACEMENT_3D('',#24236,#19478,#19479);
#17934=AXIS2_PLACEMENT_3D('',#24238,#19480,#19481);
#17935=AXIS2_PLACEMENT_3D('',#24240,#19482,#19483);
#17936=AXIS2_PLACEMENT_3D('',#24242,#19484,#19485);
#17937=AXIS2_PLACEMENT_3D('',#24244,#19486,#19487);
#17938=AXIS2_PLACEMENT_3D('',#24246,#19488,#19489);
#17939=AXIS2_PLACEMENT_3D('',#24248,#19490,#19491);
#17940=AXIS2_PLACEMENT_3D('',#24250,#19492,#19493);
#17941=AXIS2_PLACEMENT_3D('',#24252,#19494,#19495);
#17942=AXIS2_PLACEMENT_3D('',#24254,#19496,#19497);
#17943=AXIS2_PLACEMENT_3D('',#24256,#19498,#19499);
#17944=AXIS2_PLACEMENT_3D('',#24465,#19604,#19605);
#17945=AXIS2_PLACEMENT_3D('',#24683,#19714,#19715);
#17946=AXIS2_PLACEMENT_3D('',#24685,#19716,#19717);
#17947=AXIS2_PLACEMENT_3D('',#24687,#19718,#19719);
#17948=AXIS2_PLACEMENT_3D('',#24689,#19720,#19721);
#17949=AXIS2_PLACEMENT_3D('',#24691,#19722,#19723);
#17950=AXIS2_PLACEMENT_3D('',#24693,#19724,#19725);
#17951=AXIS2_PLACEMENT_3D('',#24695,#19726,#19727);
#17952=AXIS2_PLACEMENT_3D('',#24697,#19728,#19729);
#17953=AXIS2_PLACEMENT_3D('',#24699,#19730,#19731);
#17954=AXIS2_PLACEMENT_3D('',#24701,#19732,#19733);
#17955=AXIS2_PLACEMENT_3D('',#24703,#19734,#19735);
#17956=AXIS2_PLACEMENT_3D('',#24705,#19736,#19737);
#17957=AXIS2_PLACEMENT_3D('',#24707,#19738,#19739);
#17958=AXIS2_PLACEMENT_3D('',#24709,#19740,#19741);
#17959=AXIS2_PLACEMENT_3D('',#24711,#19742,#19743);
#17960=AXIS2_PLACEMENT_3D('',#24713,#19744,#19745);
#17961=AXIS2_PLACEMENT_3D('',#24715,#19746,#19747);
#17962=AXIS2_PLACEMENT_3D('',#24717,#19748,#19749);
#17963=AXIS2_PLACEMENT_3D('',#24719,#19750,#19751);
#17964=AXIS2_PLACEMENT_3D('',#24721,#19752,#19753);
#17965=AXIS2_PLACEMENT_3D('',#24723,#19754,#19755);
#17966=AXIS2_PLACEMENT_3D('',#24725,#19756,#19757);
#17967=AXIS2_PLACEMENT_3D('',#24727,#19758,#19759);
#17968=AXIS2_PLACEMENT_3D('',#24729,#19760,#19761);
#17969=AXIS2_PLACEMENT_3D('',#24731,#19762,#19763);
#17970=AXIS2_PLACEMENT_3D('',#24733,#19764,#19765);
#17971=AXIS2_PLACEMENT_3D('',#24734,#19766,#19767);
#17972=AXIS2_PLACEMENT_3D('',#24737,#19770,#19771);
#17973=AXIS2_PLACEMENT_3D('',#24739,#19773,#19774);
#17974=AXIS2_PLACEMENT_3D('',#24741,#19776,#19777);
#17975=AXIS2_PLACEMENT_3D('',#24743,#19779,#19780);
#17976=AXIS2_PLACEMENT_3D('',#24745,#19782,#19783);
#17977=AXIS2_PLACEMENT_3D('',#24747,#19785,#19786);
#17978=AXIS2_PLACEMENT_3D('',#24749,#19788,#19789);
#17979=AXIS2_PLACEMENT_3D('',#24751,#19791,#19792);
#17980=AXIS2_PLACEMENT_3D('',#24753,#19794,#19795);
#17981=AXIS2_PLACEMENT_3D('',#24755,#19797,#19798);
#17982=AXIS2_PLACEMENT_3D('',#24757,#19800,#19801);
#17983=AXIS2_PLACEMENT_3D('',#24759,#19803,#19804);
#17984=AXIS2_PLACEMENT_3D('',#24761,#19806,#19807);
#17985=AXIS2_PLACEMENT_3D('',#24763,#19809,#19810);
#17986=AXIS2_PLACEMENT_3D('',#24765,#19812,#19813);
#17987=AXIS2_PLACEMENT_3D('',#24767,#19815,#19816);
#17988=AXIS2_PLACEMENT_3D('',#24769,#19818,#19819);
#17989=AXIS2_PLACEMENT_3D('',#24771,#19821,#19822);
#17990=AXIS2_PLACEMENT_3D('',#24773,#19824,#19825);
#17991=AXIS2_PLACEMENT_3D('',#24775,#19827,#19828);
#17992=AXIS2_PLACEMENT_3D('',#24777,#19830,#19831);
#17993=AXIS2_PLACEMENT_3D('',#24779,#19833,#19834);
#17994=AXIS2_PLACEMENT_3D('',#24781,#19836,#19837);
#17995=AXIS2_PLACEMENT_3D('',#24783,#19839,#19840);
#17996=AXIS2_PLACEMENT_3D('',#24785,#19842,#19843);
#17997=AXIS2_PLACEMENT_3D('',#24787,#19845,#19846);
#17998=AXIS2_PLACEMENT_3D('',#24789,#19848,#19849);
#17999=AXIS2_PLACEMENT_3D('',#24792,#19852,#19853);
#18000=AXIS2_PLACEMENT_3D('',#24795,#19856,#19857);
#18001=AXIS2_PLACEMENT_3D('',#24798,#19860,#19861);
#18002=AXIS2_PLACEMENT_3D('',#24801,#19864,#19865);
#18003=AXIS2_PLACEMENT_3D('',#24804,#19868,#19869);
#18004=AXIS2_PLACEMENT_3D('',#24807,#19872,#19873);
#18005=AXIS2_PLACEMENT_3D('',#24810,#19876,#19877);
#18006=AXIS2_PLACEMENT_3D('',#24813,#19880,#19881);
#18007=AXIS2_PLACEMENT_3D('',#24816,#19884,#19885);
#18008=AXIS2_PLACEMENT_3D('',#24819,#19888,#19889);
#18009=AXIS2_PLACEMENT_3D('',#24822,#19892,#19893);
#18010=AXIS2_PLACEMENT_3D('',#24825,#19896,#19897);
#18011=AXIS2_PLACEMENT_3D('',#24828,#19900,#19901);
#18012=AXIS2_PLACEMENT_3D('',#24831,#19904,#19905);
#18013=AXIS2_PLACEMENT_3D('',#24834,#19908,#19909);
#18014=AXIS2_PLACEMENT_3D('',#24837,#19912,#19913);
#18015=AXIS2_PLACEMENT_3D('',#24840,#19916,#19917);
#18016=AXIS2_PLACEMENT_3D('',#24843,#19920,#19921);
#18017=AXIS2_PLACEMENT_3D('',#24846,#19924,#19925);
#18018=AXIS2_PLACEMENT_3D('',#24849,#19928,#19929);
#18019=AXIS2_PLACEMENT_3D('',#24852,#19932,#19933);
#18020=AXIS2_PLACEMENT_3D('',#24855,#19936,#19937);
#18021=AXIS2_PLACEMENT_3D('',#24858,#19940,#19941);
#18022=AXIS2_PLACEMENT_3D('',#24861,#19944,#19945);
#18023=AXIS2_PLACEMENT_3D('',#24864,#19948,#19949);
#18024=AXIS2_PLACEMENT_3D('',#24867,#19952,#19953);
#18025=AXIS2_PLACEMENT_3D('',#24869,#19955,#19956);
#18026=AXIS2_PLACEMENT_3D('',#24871,#19958,#19959);
#18027=AXIS2_PLACEMENT_3D('',#24873,#19961,#19962);
#18028=AXIS2_PLACEMENT_3D('',#24875,#19964,#19965);
#18029=AXIS2_PLACEMENT_3D('',#24876,#19966,#19967);
#18030=AXIS2_PLACEMENT_3D('',#24878,#19969,#19970);
#18031=AXIS2_PLACEMENT_3D('',#24880,#19972,#19973);
#18032=AXIS2_PLACEMENT_3D('',#24881,#19974,#19975);
#18033=AXIS2_PLACEMENT_3D('',#24883,#19977,#19978);
#18034=AXIS2_PLACEMENT_3D('',#24885,#19980,#19981);
#18035=AXIS2_PLACEMENT_3D('',#24886,#19982,#19983);
#18036=AXIS2_PLACEMENT_3D('',#24888,#19985,#19986);
#18037=AXIS2_PLACEMENT_3D('',#24890,#19988,#19989);
#18038=AXIS2_PLACEMENT_3D('',#24891,#19990,#19991);
#18039=AXIS2_PLACEMENT_3D('',#24893,#19993,#19994);
#18040=AXIS2_PLACEMENT_3D('',#24895,#19996,#19997);
#18041=AXIS2_PLACEMENT_3D('',#24896,#19998,#19999);
#18042=AXIS2_PLACEMENT_3D('',#24898,#20001,#20002);
#18043=AXIS2_PLACEMENT_3D('',#24900,#20004,#20005);
#18044=AXIS2_PLACEMENT_3D('',#24901,#20006,#20007);
#18045=AXIS2_PLACEMENT_3D('',#24903,#20009,#20010);
#18046=AXIS2_PLACEMENT_3D('',#24905,#20012,#20013);
#18047=AXIS2_PLACEMENT_3D('',#24906,#20014,#20015);
#18048=AXIS2_PLACEMENT_3D('',#24908,#20017,#20018);
#18049=AXIS2_PLACEMENT_3D('',#24910,#20020,#20021);
#18050=AXIS2_PLACEMENT_3D('',#24911,#20022,#20023);
#18051=AXIS2_PLACEMENT_3D('',#24913,#20025,#20026);
#18052=AXIS2_PLACEMENT_3D('',#24915,#20028,#20029);
#18053=AXIS2_PLACEMENT_3D('',#24916,#20030,#20031);
#18054=AXIS2_PLACEMENT_3D('',#24918,#20033,#20034);
#18055=AXIS2_PLACEMENT_3D('',#24920,#20036,#20037);
#18056=AXIS2_PLACEMENT_3D('',#24921,#20038,#20039);
#18057=AXIS2_PLACEMENT_3D('',#24923,#20041,#20042);
#18058=AXIS2_PLACEMENT_3D('',#24925,#20044,#20045);
#18059=AXIS2_PLACEMENT_3D('',#24926,#20046,#20047);
#18060=AXIS2_PLACEMENT_3D('',#24928,#20049,#20050);
#18061=AXIS2_PLACEMENT_3D('',#24930,#20052,#20053);
#18062=AXIS2_PLACEMENT_3D('',#24931,#20054,#20055);
#18063=AXIS2_PLACEMENT_3D('',#24933,#20057,#20058);
#18064=AXIS2_PLACEMENT_3D('',#24935,#20060,#20061);
#18065=AXIS2_PLACEMENT_3D('',#24936,#20062,#20063);
#18066=AXIS2_PLACEMENT_3D('',#24938,#20065,#20066);
#18067=AXIS2_PLACEMENT_3D('',#24940,#20068,#20069);
#18068=AXIS2_PLACEMENT_3D('',#24941,#20070,#20071);
#18069=AXIS2_PLACEMENT_3D('',#24943,#20073,#20074);
#18070=AXIS2_PLACEMENT_3D('',#24945,#20076,#20077);
#18071=AXIS2_PLACEMENT_3D('',#24946,#20078,#20079);
#18072=AXIS2_PLACEMENT_3D('',#24948,#20081,#20082);
#18073=AXIS2_PLACEMENT_3D('',#24950,#20084,#20085);
#18074=AXIS2_PLACEMENT_3D('',#24951,#20086,#20087);
#18075=AXIS2_PLACEMENT_3D('',#24953,#20089,#20090);
#18076=AXIS2_PLACEMENT_3D('',#24955,#20092,#20093);
#18077=AXIS2_PLACEMENT_3D('',#24956,#20094,#20095);
#18078=AXIS2_PLACEMENT_3D('',#24958,#20097,#20098);
#18079=AXIS2_PLACEMENT_3D('',#24960,#20100,#20101);
#18080=AXIS2_PLACEMENT_3D('',#24961,#20102,#20103);
#18081=AXIS2_PLACEMENT_3D('',#24963,#20105,#20106);
#18082=AXIS2_PLACEMENT_3D('',#24965,#20108,#20109);
#18083=AXIS2_PLACEMENT_3D('',#24966,#20110,#20111);
#18084=AXIS2_PLACEMENT_3D('',#24968,#20113,#20114);
#18085=AXIS2_PLACEMENT_3D('',#24970,#20116,#20117);
#18086=AXIS2_PLACEMENT_3D('',#24971,#20118,#20119);
#18087=AXIS2_PLACEMENT_3D('',#24973,#20121,#20122);
#18088=AXIS2_PLACEMENT_3D('',#24975,#20124,#20125);
#18089=AXIS2_PLACEMENT_3D('',#24976,#20126,#20127);
#18090=AXIS2_PLACEMENT_3D('',#24978,#20129,#20130);
#18091=AXIS2_PLACEMENT_3D('',#24980,#20132,#20133);
#18092=AXIS2_PLACEMENT_3D('',#24981,#20134,#20135);
#18093=AXIS2_PLACEMENT_3D('',#24983,#20137,#20138);
#18094=AXIS2_PLACEMENT_3D('',#24985,#20140,#20141);
#18095=AXIS2_PLACEMENT_3D('',#24986,#20142,#20143);
#18096=AXIS2_PLACEMENT_3D('',#24988,#20145,#20146);
#18097=AXIS2_PLACEMENT_3D('',#24990,#20148,#20149);
#18098=AXIS2_PLACEMENT_3D('',#24991,#20150,#20151);
#18099=AXIS2_PLACEMENT_3D('',#24993,#20153,#20154);
#18100=AXIS2_PLACEMENT_3D('',#24995,#20156,#20157);
#18101=AXIS2_PLACEMENT_3D('',#24996,#20158,#20159);
#18102=AXIS2_PLACEMENT_3D('',#24998,#20161,#20162);
#18103=AXIS2_PLACEMENT_3D('',#25000,#20164,#20165);
#18104=AXIS2_PLACEMENT_3D('',#25001,#20166,#20167);
#19440=DIRECTION('axis',(0.,0.,1.));
#19441=DIRECTION('refdir',(1.,0.,0.));
#19442=DIRECTION('center_axis',(-1.E-14,-1.,0.));
#19443=DIRECTION('ref_axis',(1.,-1.E-14,1.E-14));
#19444=DIRECTION('',(0.,0.,-1.));
#19445=DIRECTION('',(1.,-1.E-14,1.E-14));
#19446=DIRECTION('',(-1.E-14,0.,1.));
#19447=DIRECTION('',(1.,-1.E-14,1.E-14));
#19448=DIRECTION('center_axis',(-1.E-14,-1.,0.));
#19449=DIRECTION('ref_axis',(1.,-1.E-14,0.));
#19450=DIRECTION('center_axis',(-1.E-14,-1.,0.));
#19451=DIRECTION('ref_axis',(1.,-1.E-14,0.));
#19452=DIRECTION('center_axis',(-1.E-14,-1.,0.));
#19453=DIRECTION('ref_axis',(1.,-1.E-14,0.));
#19454=DIRECTION('center_axis',(-1.E-14,-1.,0.));
#19455=DIRECTION('ref_axis',(1.,-1.E-14,0.));
#19456=DIRECTION('center_axis',(-1.E-14,-1.,0.));
#19457=DIRECTION('ref_axis',(1.,-1.E-14,0.));
#19458=DIRECTION('center_axis',(-1.E-14,-1.,0.));
#19459=DIRECTION('ref_axis',(1.,-1.E-14,0.));
#19460=DIRECTION('center_axis',(-1.E-14,-1.,0.));
#19461=DIRECTION('ref_axis',(1.,-1.E-14,0.));
#19462=DIRECTION('center_axis',(-1.E-14,-1.,0.));
#19463=DIRECTION('ref_axis',(1.,-1.E-14,0.));
#19464=DIRECTION('center_axis',(-1.E-14,-1.,0.));
#19465=DIRECTION('ref_axis',(1.,-1.E-14,0.));
#19466=DIRECTION('center_axis',(-1.E-14,-1.,0.));
#19467=DIRECTION('ref_axis',(1.,-1.E-14,0.));
#19468=DIRECTION('center_axis',(-1.E-14,-1.,0.));
#19469=DIRECTION('ref_axis',(1.,-1.E-14,0.));
#19470=DIRECTION('center_axis',(-1.E-14,-1.,0.));
#19471=DIRECTION('ref_axis',(1.,-1.E-14,0.));
#19472=DIRECTION('center_axis',(-1.E-14,-1.,0.));
#19473=DIRECTION('ref_axis',(1.,-1.E-14,0.));
#19474=DIRECTION('center_axis',(-1.E-14,-1.,0.));
#19475=DIRECTION('ref_axis',(1.,-1.E-14,0.));
#19476=DIRECTION('center_axis',(-1.E-14,-1.,0.));
#19477=DIRECTION('ref_axis',(1.,-1.E-14,0.));
#19478=DIRECTION('center_axis',(-1.E-14,-1.,0.));
#19479=DIRECTION('ref_axis',(1.,-1.E-14,0.));
#19480=DIRECTION('center_axis',(-1.E-14,-1.,0.));
#19481=DIRECTION('ref_axis',(1.,-1.E-14,0.));
#19482=DIRECTION('center_axis',(-1.E-14,-1.,0.));
#19483=DIRECTION('ref_axis',(1.,-1.E-14,0.));
#19484=DIRECTION('center_axis',(-1.E-14,-1.,0.));
#19485=DIRECTION('ref_axis',(1.,-1.E-14,0.));
#19486=DIRECTION('center_axis',(-1.E-14,-1.,0.));
#19487=DIRECTION('ref_axis',(1.,-1.E-14,0.));
#19488=DIRECTION('center_axis',(-1.E-14,-1.,0.));
#19489=DIRECTION('ref_axis',(1.,-1.E-14,0.));
#19490=DIRECTION('center_axis',(-1.E-14,-1.,0.));
#19491=DIRECTION('ref_axis',(1.,-1.E-14,0.));
#19492=DIRECTION('center_axis',(-1.E-14,-1.,0.));
#19493=DIRECTION('ref_axis',(1.,-1.E-14,0.));
#19494=DIRECTION('center_axis',(-1.E-14,-1.,0.));
#19495=DIRECTION('ref_axis',(1.,-1.E-14,0.));
#19496=DIRECTION('center_axis',(-1.E-14,-1.,0.));
#19497=DIRECTION('ref_axis',(1.,-1.E-14,0.));
#19498=DIRECTION('center_axis',(-1.E-14,-1.,0.));
#19499=DIRECTION('ref_axis',(1.,-1.E-14,0.));
#19500=DIRECTION('',(1.,-1.E-14,1.E-14));
#19501=DIRECTION('',(-1.E-14,0.,1.));
#19502=DIRECTION('',(1.,-1.E-14,9.60574466455073E-15));
#19503=DIRECTION('',(-1.E-14,0.,1.));
#19504=DIRECTION('',(1.,-1.E-14,1.E-14));
#19505=DIRECTION('',(-1.1020425574104E-14,1.020425574104E-29,1.));
#19506=DIRECTION('',(1.,-1.E-14,9.60574466455073E-15));
#19507=DIRECTION('',(-1.E-14,0.,1.));
#19508=DIRECTION('',(1.,-1.E-14,1.E-14));
#19509=DIRECTION('',(-1.1020425574104E-14,1.020425574104E-29,1.));
#19510=DIRECTION('',(1.,-1.E-14,9.60574466455073E-15));
#19511=DIRECTION('',(-1.E-14,0.,1.));
#19512=DIRECTION('',(1.,-1.E-14,1.E-14));
#19513=DIRECTION('',(-1.E-14,0.,1.));
#19514=DIRECTION('',(1.,-1.E-14,9.60574466455073E-15));
#19515=DIRECTION('',(-1.E-14,0.,1.));
#19516=DIRECTION('',(1.,-1.E-14,1.E-14));
#19517=DIRECTION('',(-1.E-14,0.,1.));
#19518=DIRECTION('',(1.,-1.E-14,9.60574466455073E-15));
#19519=DIRECTION('',(-1.E-14,0.,1.));
#19520=DIRECTION('',(1.,-1.E-14,1.E-14));
#19521=DIRECTION('',(-1.E-14,0.,1.));
#19522=DIRECTION('',(1.,-1.E-14,9.60574466455073E-15));
#19523=DIRECTION('',(-1.E-14,0.,1.));
#19524=DIRECTION('',(1.,-1.E-14,1.E-14));
#19525=DIRECTION('',(-1.E-14,0.,1.));
#19526=DIRECTION('',(1.,-1.E-14,9.60574466455073E-15));
#19527=DIRECTION('',(-1.E-14,0.,1.));
#19528=DIRECTION('',(1.,-1.E-14,1.E-14));
#19529=DIRECTION('',(-1.E-14,0.,1.));
#19530=DIRECTION('',(1.,-1.E-14,9.60574466455073E-15));
#19531=DIRECTION('',(-1.E-14,0.,1.));
#19532=DIRECTION('',(1.,-1.E-14,1.E-14));
#19533=DIRECTION('',(-1.E-14,0.,1.));
#19534=DIRECTION('',(1.,-1.E-14,9.60574466455073E-15));
#19535=DIRECTION('',(-1.E-14,0.,1.));
#19536=DIRECTION('',(1.,-1.E-14,1.E-14));
#19537=DIRECTION('',(-1.E-14,0.,1.));
#19538=DIRECTION('',(1.,-1.E-14,9.60574466455073E-15));
#19539=DIRECTION('',(-1.E-14,0.,1.));
#19540=DIRECTION('',(1.,-1.E-14,1.E-14));
#19541=DIRECTION('',(-1.E-14,0.,1.));
#19542=DIRECTION('',(1.,-1.E-14,9.60574466455073E-15));
#19543=DIRECTION('',(-1.E-14,0.,1.));
#19544=DIRECTION('',(1.,-1.E-14,1.E-14));
#19545=DIRECTION('',(-1.E-14,0.,1.));
#19546=DIRECTION('',(1.,-1.E-14,9.60574466455073E-15));
#19547=DIRECTION('',(-1.E-14,0.,1.));
#19548=DIRECTION('',(1.,-1.E-14,1.E-14));
#19549=DIRECTION('',(-1.E-14,0.,1.));
#19550=DIRECTION('',(1.,-1.E-14,9.60574466455073E-15));
#19551=DIRECTION('',(-1.E-14,0.,1.));
#19552=DIRECTION('',(1.,-1.E-14,1.E-14));
#19553=DIRECTION('',(-1.E-14,0.,1.));
#19554=DIRECTION('',(1.,-1.E-14,9.60574466455073E-15));
#19555=DIRECTION('',(-1.E-14,0.,1.));
#19556=DIRECTION('',(1.,-1.E-14,1.E-14));
#19557=DIRECTION('',(-1.E-14,0.,1.));
#19558=DIRECTION('',(1.,-1.E-14,9.60574466455073E-15));
#19559=DIRECTION('',(-1.E-14,0.,1.));
#19560=DIRECTION('',(1.,-1.E-14,1.E-14));
#19561=DIRECTION('',(-1.E-14,0.,1.));
#19562=DIRECTION('',(1.,-1.E-14,9.60574466455073E-15));
#19563=DIRECTION('',(-1.E-14,0.,1.));
#19564=DIRECTION('',(1.,-1.E-14,1.E-14));
#19565=DIRECTION('',(-1.E-14,0.,1.));
#19566=DIRECTION('',(1.,-1.E-14,9.60574466455073E-15));
#19567=DIRECTION('',(-1.E-14,0.,1.));
#19568=DIRECTION('',(1.,-1.E-14,1.E-14));
#19569=DIRECTION('',(-1.E-14,0.,1.));
#19570=DIRECTION('',(1.,-1.E-14,9.60574466455073E-15));
#19571=DIRECTION('',(-1.E-14,0.,1.));
#19572=DIRECTION('',(1.,-1.E-14,1.E-14));
#19573=DIRECTION('',(-1.E-14,0.,1.));
#19574=DIRECTION('',(1.,-1.E-14,9.60574466455073E-15));
#19575=DIRECTION('',(-1.E-14,0.,1.));
#19576=DIRECTION('',(1.,-1.E-14,1.E-14));
#19577=DIRECTION('',(-1.E-14,0.,1.));
#19578=DIRECTION('',(1.,-1.E-14,9.60574466455073E-15));
#19579=DIRECTION('',(-1.E-14,0.,1.));
#19580=DIRECTION('',(1.,-1.E-14,1.E-14));
#19581=DIRECTION('',(-1.E-14,0.,1.));
#19582=DIRECTION('',(1.,-1.E-14,9.60574466455073E-15));
#19583=DIRECTION('',(-1.E-14,0.,1.));
#19584=DIRECTION('',(1.,-1.E-14,1.E-14));
#19585=DIRECTION('',(-1.E-14,0.,1.));
#19586=DIRECTION('',(1.,-1.E-14,9.60574466455073E-15));
#19587=DIRECTION('',(-1.E-14,0.,1.));
#19588=DIRECTION('',(1.,-1.E-14,1.E-14));
#19589=DIRECTION('',(-1.E-14,0.,1.));
#19590=DIRECTION('',(1.,-1.E-14,9.60574466455073E-15));
#19591=DIRECTION('',(-1.E-14,0.,1.));
#19592=DIRECTION('',(1.,-1.E-14,1.E-14));
#19593=DIRECTION('',(-1.E-14,0.,1.));
#19594=DIRECTION('',(1.,-1.E-14,9.60574466455073E-15));
#19595=DIRECTION('',(-1.E-14,0.,1.));
#19596=DIRECTION('',(1.,-1.E-14,1.E-14));
#19597=DIRECTION('',(-1.E-14,0.,1.));
#19598=DIRECTION('',(1.,-1.E-14,9.60574466455073E-15));
#19599=DIRECTION('',(-1.E-14,0.,1.));
#19600=DIRECTION('',(1.,-1.E-14,1.E-14));
#19601=DIRECTION('',(-1.E-14,0.,1.));
#19602=DIRECTION('',(1.,-1.E-14,9.60574466455073E-15));
#19603=DIRECTION('',(-1.E-14,0.,1.));
#19604=DIRECTION('center_axis',(-1.E-14,-1.,0.));
#19605=DIRECTION('ref_axis',(1.,-1.E-14,1.E-14));
#19606=DIRECTION('',(0.,0.,1.));
#19607=DIRECTION('',(1.,-1.E-14,1.E-14));
#19608=DIRECTION('',(-1.E-14,0.,1.));
#19609=DIRECTION('',(1.,-1.E-14,1.E-14));
#19610=DIRECTION('',(1.,-1.E-14,1.E-14));
#19611=DIRECTION('',(-1.E-14,0.,1.));
#19612=DIRECTION('',(1.,-1.E-14,9.60574466455073E-15));
#19613=DIRECTION('',(-1.E-14,0.,1.));
#19614=DIRECTION('',(1.,-1.E-14,1.E-14));
#19615=DIRECTION('',(-1.E-14,0.,1.));
#19616=DIRECTION('',(1.,-1.E-14,9.60574466455073E-15));
#19617=DIRECTION('',(-1.E-14,0.,1.));
#19618=DIRECTION('',(1.,-1.E-14,1.E-14));
#19619=DIRECTION('',(-1.E-14,0.,1.));
#19620=DIRECTION('',(1.,-1.E-14,9.60574466455073E-15));
#19621=DIRECTION('',(-1.E-14,0.,1.));
#19622=DIRECTION('',(1.,-1.E-14,1.E-14));
#19623=DIRECTION('',(-1.E-14,0.,1.));
#19624=DIRECTION('',(1.,-1.E-14,9.60574466455073E-15));
#19625=DIRECTION('',(-1.E-14,0.,1.));
#19626=DIRECTION('',(1.,-1.E-14,1.E-14));
#19627=DIRECTION('',(-1.E-14,0.,1.));
#19628=DIRECTION('',(1.,-1.E-14,9.60574466455073E-15));
#19629=DIRECTION('',(-1.E-14,0.,1.));
#19630=DIRECTION('',(1.,-1.E-14,1.E-14));
#19631=DIRECTION('',(-1.E-14,0.,1.));
#19632=DIRECTION('',(1.,-1.E-14,9.60574466455073E-15));
#19633=DIRECTION('',(-1.E-14,0.,1.));
#19634=DIRECTION('',(1.,-1.E-14,1.E-14));
#19635=DIRECTION('',(-1.E-14,0.,1.));
#19636=DIRECTION('',(1.,-1.E-14,9.60574466455073E-15));
#19637=DIRECTION('',(-1.E-14,0.,1.));
#19638=DIRECTION('',(1.,-1.E-14,1.E-14));
#19639=DIRECTION('',(-1.E-14,0.,1.));
#19640=DIRECTION('',(1.,-1.E-14,9.60574466455073E-15));
#19641=DIRECTION('',(-1.E-14,0.,1.));
#19642=DIRECTION('',(1.,-1.E-14,1.E-14));
#19643=DIRECTION('',(-1.E-14,0.,1.));
#19644=DIRECTION('',(1.,-1.E-14,9.60574466455073E-15));
#19645=DIRECTION('',(-1.E-14,0.,1.));
#19646=DIRECTION('',(1.,-1.E-14,1.E-14));
#19647=DIRECTION('',(-1.E-14,0.,1.));
#19648=DIRECTION('',(1.,-1.E-14,9.60574466455073E-15));
#19649=DIRECTION('',(-1.E-14,0.,1.));
#19650=DIRECTION('',(1.,-1.E-14,1.E-14));
#19651=DIRECTION('',(-1.E-14,0.,1.));
#19652=DIRECTION('',(1.,-1.E-14,9.60574466455073E-15));
#19653=DIRECTION('',(-1.E-14,0.,1.));
#19654=DIRECTION('',(1.,-1.E-14,1.E-14));
#19655=DIRECTION('',(-1.E-14,0.,1.));
#19656=DIRECTION('',(1.,-1.E-14,9.60574466455073E-15));
#19657=DIRECTION('',(-1.E-14,0.,1.));
#19658=DIRECTION('',(1.,-1.E-14,1.E-14));
#19659=DIRECTION('',(-1.E-14,0.,1.));
#19660=DIRECTION('',(1.,-1.E-14,9.60574466455073E-15));
#19661=DIRECTION('',(-1.E-14,0.,1.));
#19662=DIRECTION('',(1.,-1.E-14,1.E-14));
#19663=DIRECTION('',(-1.E-14,0.,1.));
#19664=DIRECTION('',(1.,-1.E-14,9.60574466455073E-15));
#19665=DIRECTION('',(-1.E-14,0.,1.));
#19666=DIRECTION('',(1.,-1.E-14,1.E-14));
#19667=DIRECTION('',(-1.E-14,0.,1.));
#19668=DIRECTION('',(1.,-1.E-14,9.60574466455073E-15));
#19669=DIRECTION('',(-1.E-14,0.,1.));
#19670=DIRECTION('',(1.,-1.E-14,1.E-14));
#19671=DIRECTION('',(-1.E-14,0.,1.));
#19672=DIRECTION('',(1.,-1.E-14,9.60574466455073E-15));
#19673=DIRECTION('',(-1.E-14,0.,1.));
#19674=DIRECTION('',(1.,-1.E-14,1.E-14));
#19675=DIRECTION('',(-1.E-14,0.,1.));
#19676=DIRECTION('',(1.,-1.E-14,9.60574466455073E-15));
#19677=DIRECTION('',(-1.E-14,0.,1.));
#19678=DIRECTION('',(1.,-1.E-14,1.E-14));
#19679=DIRECTION('',(-1.E-14,0.,1.));
#19680=DIRECTION('',(1.,-1.E-14,9.60574466455073E-15));
#19681=DIRECTION('',(-1.E-14,0.,1.));
#19682=DIRECTION('',(1.,-1.E-14,1.E-14));
#19683=DIRECTION('',(-1.E-14,0.,1.));
#19684=DIRECTION('',(1.,-1.E-14,9.60574466455073E-15));
#19685=DIRECTION('',(-1.E-14,0.,1.));
#19686=DIRECTION('',(1.,-1.E-14,1.E-14));
#19687=DIRECTION('',(-1.E-14,0.,1.));
#19688=DIRECTION('',(1.,-1.E-14,9.60574466455073E-15));
#19689=DIRECTION('',(-1.E-14,0.,1.));
#19690=DIRECTION('',(1.,-1.E-14,1.E-14));
#19691=DIRECTION('',(-1.E-14,0.,1.));
#19692=DIRECTION('',(1.,-1.E-14,9.60574466455073E-15));
#19693=DIRECTION('',(-1.E-14,0.,1.));
#19694=DIRECTION('',(1.,-1.E-14,1.E-14));
#19695=DIRECTION('',(-1.E-14,0.,1.));
#19696=DIRECTION('',(1.,-1.E-14,9.60574466455073E-15));
#19697=DIRECTION('',(-1.E-14,0.,1.));
#19698=DIRECTION('',(1.,-1.E-14,1.E-14));
#19699=DIRECTION('',(-1.E-14,0.,1.));
#19700=DIRECTION('',(1.,-1.E-14,9.60574466455073E-15));
#19701=DIRECTION('',(-1.E-14,0.,1.));
#19702=DIRECTION('',(1.,-1.E-14,1.E-14));
#19703=DIRECTION('',(-1.E-14,0.,1.));
#19704=DIRECTION('',(1.,-1.E-14,9.60574466455073E-15));
#19705=DIRECTION('',(-1.1020425574104E-14,1.020425574104E-29,1.));
#19706=DIRECTION('',(1.,-1.E-14,1.E-14));
#19707=DIRECTION('',(-1.E-14,0.,1.));
#19708=DIRECTION('',(1.,-1.E-14,9.60574466455073E-15));
#19709=DIRECTION('',(-1.1020425574104E-14,1.020425574104E-29,1.));
#19710=DIRECTION('',(1.,-1.E-14,1.E-14));
#19711=DIRECTION('',(-1.E-14,0.,1.));
#19712=DIRECTION('',(1.,-1.E-14,9.60574466455073E-15));
#19713=DIRECTION('',(-1.E-14,0.,1.));
#19714=DIRECTION('center_axis',(-1.E-14,-1.,0.));
#19715=DIRECTION('ref_axis',(1.,-1.E-14,0.));
#19716=DIRECTION('center_axis',(-1.E-14,-1.,0.));
#19717=DIRECTION('ref_axis',(1.,-1.E-14,0.));
#19718=DIRECTION('center_axis',(-1.E-14,-1.,0.));
#19719=DIRECTION('ref_axis',(1.,-1.E-14,0.));
#19720=DIRECTION('center_axis',(-1.E-14,-1.,0.));
#19721=DIRECTION('ref_axis',(1.,-1.E-14,0.));
#19722=DIRECTION('center_axis',(-1.E-14,-1.,0.));
#19723=DIRECTION('ref_axis',(1.,-1.E-14,0.));
#19724=DIRECTION('center_axis',(-1.E-14,-1.,0.));
#19725=DIRECTION('ref_axis',(1.,-1.E-14,0.));
#19726=DIRECTION('center_axis',(-1.E-14,-1.,0.));
#19727=DIRECTION('ref_axis',(1.,-1.E-14,0.));
#19728=DIRECTION('center_axis',(-1.E-14,-1.,0.));
#19729=DIRECTION('ref_axis',(1.,-1.E-14,0.));
#19730=DIRECTION('center_axis',(-1.E-14,-1.,0.));
#19731=DIRECTION('ref_axis',(1.,-1.E-14,0.));
#19732=DIRECTION('center_axis',(-1.E-14,-1.,0.));
#19733=DIRECTION('ref_axis',(1.,-1.E-14,0.));
#19734=DIRECTION('center_axis',(-1.E-14,-1.,0.));
#19735=DIRECTION('ref_axis',(1.,-1.E-14,0.));
#19736=DIRECTION('center_axis',(-1.E-14,-1.,0.));
#19737=DIRECTION('ref_axis',(1.,-1.E-14,0.));
#19738=DIRECTION('center_axis',(-1.E-14,-1.,0.));
#19739=DIRECTION('ref_axis',(1.,-1.E-14,0.));
#19740=DIRECTION('center_axis',(-1.E-14,-1.,0.));
#19741=DIRECTION('ref_axis',(1.,-1.E-14,0.));
#19742=DIRECTION('center_axis',(-1.E-14,-1.,0.));
#19743=DIRECTION('ref_axis',(1.,-1.E-14,0.));
#19744=DIRECTION('center_axis',(-1.E-14,-1.,0.));
#19745=DIRECTION('ref_axis',(1.,-1.E-14,0.));
#19746=DIRECTION('center_axis',(-1.E-14,-1.,0.));
#19747=DIRECTION('ref_axis',(1.,-1.E-14,0.));
#19748=DIRECTION('center_axis',(-1.E-14,-1.,0.));
#19749=DIRECTION('ref_axis',(1.,-1.E-14,0.));
#19750=DIRECTION('center_axis',(-1.E-14,-1.,0.));
#19751=DIRECTION('ref_axis',(1.,-1.E-14,0.));
#19752=DIRECTION('center_axis',(-1.E-14,-1.,0.));
#19753=DIRECTION('ref_axis',(1.,-1.E-14,0.));
#19754=DIRECTION('center_axis',(-1.E-14,-1.,0.));
#19755=DIRECTION('ref_axis',(1.,-1.E-14,0.));
#19756=DIRECTION('center_axis',(-1.E-14,-1.,0.));
#19757=DIRECTION('ref_axis',(1.,-1.E-14,0.));
#19758=DIRECTION('center_axis',(-1.E-14,-1.,0.));
#19759=DIRECTION('ref_axis',(1.,-1.E-14,0.));
#19760=DIRECTION('center_axis',(-1.E-14,-1.,0.));
#19761=DIRECTION('ref_axis',(1.,-1.E-14,0.));
#19762=DIRECTION('center_axis',(-1.E-14,-1.,0.));
#19763=DIRECTION('ref_axis',(1.,-1.E-14,0.));
#19764=DIRECTION('center_axis',(-1.E-14,-1.,0.));
#19765=DIRECTION('ref_axis',(1.,-1.E-14,0.));
#19766=DIRECTION('center_axis',(-1.,1.E-14,-1.E-14));
#19767=DIRECTION('ref_axis',(-1.E-14,-1.,-2.64060752475192E-45));
#19768=DIRECTION('',(1.E-14,1.,0.));
#19769=DIRECTION('',(1.E-14,1.,0.));
#19770=DIRECTION('center_axis',(1.E-14,1.,0.));
#19771=DIRECTION('ref_axis',(-1.,1.E-14,0.));
#19772=DIRECTION('',(1.E-14,1.,0.));
#19773=DIRECTION('center_axis',(1.E-14,1.,0.));
#19774=DIRECTION('ref_axis',(-1.,1.E-14,0.));
#19775=DIRECTION('',(1.E-14,1.,0.));
#19776=DIRECTION('center_axis',(1.E-14,1.,0.));
#19777=DIRECTION('ref_axis',(-1.,1.E-14,0.));
#19778=DIRECTION('',(1.E-14,1.,0.));
#19779=DIRECTION('center_axis',(1.E-14,1.,0.));
#19780=DIRECTION('ref_axis',(-1.,1.E-14,0.));
#19781=DIRECTION('',(1.E-14,1.,0.));
#19782=DIRECTION('center_axis',(1.E-14,1.,0.));
#19783=DIRECTION('ref_axis',(-1.,1.E-14,0.));
#19784=DIRECTION('',(1.E-14,1.,0.));
#19785=DIRECTION('center_axis',(1.E-14,1.,0.));
#19786=DIRECTION('ref_axis',(-1.,1.E-14,0.));
#19787=DIRECTION('',(1.E-14,1.,0.));
#19788=DIRECTION('center_axis',(1.E-14,1.,0.));
#19789=DIRECTION('ref_axis',(-1.,1.E-14,0.));
#19790=DIRECTION('',(1.E-14,1.,0.));
#19791=DIRECTION('center_axis',(1.E-14,1.,0.));
#19792=DIRECTION('ref_axis',(-1.,1.E-14,0.));
#19793=DIRECTION('',(1.E-14,1.,0.));
#19794=DIRECTION('center_axis',(1.E-14,1.,0.));
#19795=DIRECTION('ref_axis',(-1.,1.E-14,0.));
#19796=DIRECTION('',(1.E-14,1.,0.));
#19797=DIRECTION('center_axis',(1.E-14,1.,0.));
#19798=DIRECTION('ref_axis',(-1.,1.E-14,0.));
#19799=DIRECTION('',(1.E-14,1.,0.));
#19800=DIRECTION('center_axis',(1.E-14,1.,0.));
#19801=DIRECTION('ref_axis',(-1.,1.E-14,0.));
#19802=DIRECTION('',(1.E-14,1.,0.));
#19803=DIRECTION('center_axis',(1.E-14,1.,0.));
#19804=DIRECTION('ref_axis',(-1.,1.E-14,0.));
#19805=DIRECTION('',(1.E-14,1.,0.));
#19806=DIRECTION('center_axis',(1.E-14,1.,0.));
#19807=DIRECTION('ref_axis',(-1.,1.E-14,0.));
#19808=DIRECTION('',(1.E-14,1.,0.));
#19809=DIRECTION('center_axis',(1.E-14,1.,0.));
#19810=DIRECTION('ref_axis',(-1.,1.E-14,0.));
#19811=DIRECTION('',(1.E-14,1.,0.));
#19812=DIRECTION('center_axis',(1.E-14,1.,0.));
#19813=DIRECTION('ref_axis',(-1.,1.E-14,0.));
#19814=DIRECTION('',(1.E-14,1.,0.));
#19815=DIRECTION('center_axis',(1.E-14,1.,0.));
#19816=DIRECTION('ref_axis',(-1.,1.E-14,0.));
#19817=DIRECTION('',(1.E-14,1.,0.));
#19818=DIRECTION('center_axis',(1.E-14,1.,0.));
#19819=DIRECTION('ref_axis',(-1.,1.E-14,0.));
#19820=DIRECTION('',(1.E-14,1.,0.));
#19821=DIRECTION('center_axis',(1.E-14,1.,0.));
#19822=DIRECTION('ref_axis',(-1.,1.E-14,0.));
#19823=DIRECTION('',(1.E-14,1.,0.));
#19824=DIRECTION('center_axis',(1.E-14,1.,0.));
#19825=DIRECTION('ref_axis',(-1.,1.E-14,0.));
#19826=DIRECTION('',(1.E-14,1.,0.));
#19827=DIRECTION('center_axis',(1.E-14,1.,0.));
#19828=DIRECTION('ref_axis',(-1.,1.E-14,0.));
#19829=DIRECTION('',(1.E-14,1.,0.));
#19830=DIRECTION('center_axis',(1.E-14,1.,0.));
#19831=DIRECTION('ref_axis',(-1.,1.E-14,0.));
#19832=DIRECTION('',(1.E-14,1.,0.));
#19833=DIRECTION('center_axis',(1.E-14,1.,0.));
#19834=DIRECTION('ref_axis',(-1.,1.E-14,0.));
#19835=DIRECTION('',(1.E-14,1.,0.));
#19836=DIRECTION('center_axis',(1.E-14,1.,0.));
#19837=DIRECTION('ref_axis',(-1.,1.E-14,0.));
#19838=DIRECTION('',(1.E-14,1.,0.));
#19839=DIRECTION('center_axis',(1.E-14,1.,0.));
#19840=DIRECTION('ref_axis',(-1.,1.E-14,0.));
#19841=DIRECTION('',(1.E-14,1.,0.));
#19842=DIRECTION('center_axis',(1.E-14,1.,0.));
#19843=DIRECTION('ref_axis',(-1.,1.E-14,0.));
#19844=DIRECTION('',(1.E-14,1.,0.));
#19845=DIRECTION('center_axis',(1.E-14,1.,0.));
#19846=DIRECTION('ref_axis',(-1.,1.E-14,0.));
#19847=DIRECTION('',(1.E-14,1.,0.));
#19848=DIRECTION('center_axis',(-1.,1.E-14,-1.E-14));
#19849=DIRECTION('ref_axis',(-1.E-14,-1.,-2.64060752475192E-45));
#19850=DIRECTION('',(1.E-14,1.,0.));
#19851=DIRECTION('',(1.E-14,1.,0.));
#19852=DIRECTION('center_axis',(-1.,1.E-14,-1.1020425574104E-14));
#19853=DIRECTION('ref_axis',(-1.1020425574104E-14,1.020425574104E-29,1.));
#19854=DIRECTION('',(1.E-14,1.,0.));
#19855=DIRECTION('',(1.E-14,1.,0.));
#19856=DIRECTION('center_axis',(-1.,1.E-14,-1.1020425574104E-14));
#19857=DIRECTION('ref_axis',(-1.1020425574104E-14,1.020425574104E-29,1.));
#19858=DIRECTION('',(1.E-14,1.,0.));
#19859=DIRECTION('',(1.E-14,1.,0.));
#19860=DIRECTION('center_axis',(-1.,1.E-14,-1.E-14));
#19861=DIRECTION('ref_axis',(-1.E-14,-1.,-2.64060752475192E-45));
#19862=DIRECTION('',(1.E-14,1.,0.));
#19863=DIRECTION('',(1.E-14,1.,0.));
#19864=DIRECTION('center_axis',(-1.,1.E-14,-1.E-14));
#19865=DIRECTION('ref_axis',(-1.E-14,-1.,-2.64060752475192E-45));
#19866=DIRECTION('',(1.E-14,1.,0.));
#19867=DIRECTION('',(1.E-14,1.,0.));
#19868=DIRECTION('center_axis',(-1.,1.E-14,-1.E-14));
#19869=DIRECTION('ref_axis',(-1.E-14,-1.,-2.64060752475192E-45));
#19870=DIRECTION('',(1.E-14,1.,0.));
#19871=DIRECTION('',(1.E-14,1.,0.));
#19872=DIRECTION('center_axis',(-1.,1.E-14,-1.E-14));
#19873=DIRECTION('ref_axis',(-1.E-14,-1.,-2.64060752475192E-45));
#19874=DIRECTION('',(1.E-14,1.,0.));
#19875=DIRECTION('',(1.E-14,1.,0.));
#19876=DIRECTION('center_axis',(-1.,1.E-14,-1.E-14));
#19877=DIRECTION('ref_axis',(-1.E-14,-1.,-2.64060752475192E-45));
#19878=DIRECTION('',(1.E-14,1.,0.));
#19879=DIRECTION('',(1.E-14,1.,0.));
#19880=DIRECTION('center_axis',(-1.,1.E-14,-1.E-14));
#19881=DIRECTION('ref_axis',(-1.E-14,-1.,-2.64060752475192E-45));
#19882=DIRECTION('',(1.E-14,1.,0.));
#19883=DIRECTION('',(1.E-14,1.,0.));
#19884=DIRECTION('center_axis',(-1.,1.E-14,-1.E-14));
#19885=DIRECTION('ref_axis',(-1.E-14,-1.,-2.64060752475192E-45));
#19886=DIRECTION('',(1.E-14,1.,0.));
#19887=DIRECTION('',(1.E-14,1.,0.));
#19888=DIRECTION('center_axis',(-1.,1.E-14,-1.E-14));
#19889=DIRECTION('ref_axis',(-1.E-14,-1.,-2.64060752475192E-45));
#19890=DIRECTION('',(1.E-14,1.,0.));
#19891=DIRECTION('',(1.E-14,1.,0.));
#19892=DIRECTION('center_axis',(-1.,1.E-14,-1.E-14));
#19893=DIRECTION('ref_axis',(-1.E-14,-1.,-2.64060752475192E-45));
#19894=DIRECTION('',(1.E-14,1.,0.));
#19895=DIRECTION('',(1.E-14,1.,0.));
#19896=DIRECTION('center_axis',(-1.,1.E-14,-1.E-14));
#19897=DIRECTION('ref_axis',(-1.E-14,-1.,-2.64060752475192E-45));
#19898=DIRECTION('',(1.E-14,1.,0.));
#19899=DIRECTION('',(1.E-14,1.,0.));
#19900=DIRECTION('center_axis',(-1.,1.E-14,-1.E-14));
#19901=DIRECTION('ref_axis',(-1.E-14,-1.,-2.64060752475192E-45));
#19902=DIRECTION('',(1.E-14,1.,0.));
#19903=DIRECTION('',(1.E-14,1.,0.));
#19904=DIRECTION('center_axis',(-1.,1.E-14,-1.E-14));
#19905=DIRECTION('ref_axis',(-1.E-14,-1.,-2.64060752475192E-45));
#19906=DIRECTION('',(1.E-14,1.,0.));
#19907=DIRECTION('',(1.E-14,1.,0.));
#19908=DIRECTION('center_axis',(-1.,1.E-14,-1.E-14));
#19909=DIRECTION('ref_axis',(-1.E-14,-1.,-2.64060752475192E-45));
#19910=DIRECTION('',(1.E-14,1.,0.));
#19911=DIRECTION('',(1.E-14,1.,0.));
#19912=DIRECTION('center_axis',(-1.,1.E-14,-1.E-14));
#19913=DIRECTION('ref_axis',(-1.E-14,-1.,-2.64060752475192E-45));
#19914=DIRECTION('',(1.E-14,1.,0.));
#19915=DIRECTION('',(1.E-14,1.,0.));
#19916=DIRECTION('center_axis',(-1.,1.E-14,-1.E-14));
#19917=DIRECTION('ref_axis',(-1.E-14,-1.,-2.64060752475192E-45));
#19918=DIRECTION('',(1.E-14,1.,0.));
#19919=DIRECTION('',(1.E-14,1.,0.));
#19920=DIRECTION('center_axis',(-1.,1.E-14,-1.E-14));
#19921=DIRECTION('ref_axis',(-1.E-14,-1.,-2.64060752475192E-45));
#19922=DIRECTION('',(1.E-14,1.,0.));
#19923=DIRECTION('',(1.E-14,1.,0.));
#19924=DIRECTION('center_axis',(-1.,1.E-14,-1.E-14));
#19925=DIRECTION('ref_axis',(-1.E-14,-1.,-2.64060752475192E-45));
#19926=DIRECTION('',(1.E-14,1.,0.));
#19927=DIRECTION('',(1.E-14,1.,0.));
#19928=DIRECTION('center_axis',(-1.,1.E-14,-1.E-14));
#19929=DIRECTION('ref_axis',(-1.E-14,-1.,-2.64060752475192E-45));
#19930=DIRECTION('',(1.E-14,1.,0.));
#19931=DIRECTION('',(1.E-14,1.,0.));
#19932=DIRECTION('center_axis',(-1.,1.E-14,-1.E-14));
#19933=DIRECTION('ref_axis',(-1.E-14,-1.,-2.64060752475192E-45));
#19934=DIRECTION('',(1.E-14,1.,0.));
#19935=DIRECTION('',(1.E-14,1.,0.));
#19936=DIRECTION('center_axis',(-1.,1.E-14,-1.E-14));
#19937=DIRECTION('ref_axis',(-1.E-14,-1.,-2.64060752475192E-45));
#19938=DIRECTION('',(1.E-14,1.,0.));
#19939=DIRECTION('',(1.E-14,1.,0.));
#19940=DIRECTION('center_axis',(-1.,1.E-14,-1.E-14));
#19941=DIRECTION('ref_axis',(-1.E-14,-1.,-2.64060752475192E-45));
#19942=DIRECTION('',(1.E-14,1.,0.));
#19943=DIRECTION('',(1.E-14,1.,0.));
#19944=DIRECTION('center_axis',(-1.,1.E-14,-1.E-14));
#19945=DIRECTION('ref_axis',(-1.E-14,-1.,-2.64060752475192E-45));
#19946=DIRECTION('',(1.E-14,1.,0.));
#19947=DIRECTION('',(1.E-14,1.,0.));
#19948=DIRECTION('center_axis',(-1.E-14,0.,1.));
#19949=DIRECTION('ref_axis',(1.,-1.E-14,1.E-14));
#19950=DIRECTION('',(1.E-14,1.,1.E-28));
#19951=DIRECTION('',(1.E-14,1.,0.));
#19952=DIRECTION('center_axis',(-1.,1.E-14,-1.E-14));
#19953=DIRECTION('ref_axis',(-1.E-14,-1.,-2.64060752475192E-45));
#19954=DIRECTION('',(1.E-14,1.,0.));
#19955=DIRECTION('center_axis',(-1.E-14,0.,1.));
#19956=DIRECTION('ref_axis',(1.,-1.E-14,1.E-14));
#19957=DIRECTION('',(1.E-14,1.,1.E-28));
#19958=DIRECTION('center_axis',(-9.60574466455073E-15,-3.94255335449275E-30,
1.));
#19959=DIRECTION('ref_axis',(1.,-1.E-14,9.60574466455073E-15));
#19960=DIRECTION('',(1.E-14,1.,0.));
#19961=DIRECTION('center_axis',(-1.,1.E-14,-1.E-14));
#19962=DIRECTION('ref_axis',(-1.E-14,-1.,-2.64060752475192E-45));
#19963=DIRECTION('',(1.E-14,1.,0.));
#19964=DIRECTION('center_axis',(-1.E-14,0.,1.));
#19965=DIRECTION('ref_axis',(1.,-1.E-14,1.E-14));
#19966=DIRECTION('center_axis',(-9.60574466455072E-15,-3.94255335449275E-30,
1.));
#19967=DIRECTION('ref_axis',(1.,-1.E-14,9.60574466455072E-15));
#19968=DIRECTION('',(1.E-14,1.,0.));
#19969=DIRECTION('center_axis',(-1.,1.E-14,-1.E-14));
#19970=DIRECTION('ref_axis',(-1.E-14,-1.,-2.64060752475192E-45));
#19971=DIRECTION('',(1.E-14,1.,0.));
#19972=DIRECTION('center_axis',(-1.E-14,0.,1.));
#19973=DIRECTION('ref_axis',(1.,-1.E-14,1.E-14));
#19974=DIRECTION('center_axis',(-9.60574466455072E-15,-3.94255335449275E-30,
1.));
#19975=DIRECTION('ref_axis',(1.,-1.E-14,9.60574466455072E-15));
#19976=DIRECTION('',(1.E-14,1.,0.));
#19977=DIRECTION('center_axis',(-1.,1.E-14,-1.E-14));
#19978=DIRECTION('ref_axis',(-1.E-14,-1.,-2.64060752475192E-45));
#19979=DIRECTION('',(1.E-14,1.,0.));
#19980=DIRECTION('center_axis',(-1.E-14,0.,1.));
#19981=DIRECTION('ref_axis',(1.,-1.E-14,1.E-14));
#19982=DIRECTION('center_axis',(-9.60574466455073E-15,-3.94255335449275E-30,
1.));
#19983=DIRECTION('ref_axis',(1.,-1.E-14,9.60574466455073E-15));
#19984=DIRECTION('',(1.E-14,1.,0.));
#19985=DIRECTION('center_axis',(-1.,1.E-14,-1.E-14));
#19986=DIRECTION('ref_axis',(-1.E-14,-1.,-2.64060752475192E-45));
#19987=DIRECTION('',(1.E-14,1.,0.));
#19988=DIRECTION('center_axis',(-1.E-14,0.,1.));
#19989=DIRECTION('ref_axis',(1.,-1.E-14,1.E-14));
#19990=DIRECTION('center_axis',(-9.60574466455073E-15,-3.94255335449275E-30,
1.));
#19991=DIRECTION('ref_axis',(1.,-1.E-14,9.60574466455073E-15));
#19992=DIRECTION('',(1.E-14,1.,0.));
#19993=DIRECTION('center_axis',(-1.,1.E-14,-1.E-14));
#19994=DIRECTION('ref_axis',(-1.E-14,-1.,-2.64060752475192E-45));
#19995=DIRECTION('',(1.E-14,1.,0.));
#19996=DIRECTION('center_axis',(-1.E-14,0.,1.));
#19997=DIRECTION('ref_axis',(1.,-1.E-14,1.E-14));
#19998=DIRECTION('center_axis',(-9.60574466455073E-15,-3.94255335449275E-30,
1.));
#19999=DIRECTION('ref_axis',(1.,-1.E-14,9.60574466455073E-15));
#20000=DIRECTION('',(1.E-14,1.,0.));
#20001=DIRECTION('center_axis',(-1.,1.E-14,-1.E-14));
#20002=DIRECTION('ref_axis',(-1.E-14,-1.,-2.64060752475192E-45));
#20003=DIRECTION('',(1.E-14,1.,0.));
#20004=DIRECTION('center_axis',(-1.E-14,0.,1.));
#20005=DIRECTION('ref_axis',(1.,-1.E-14,1.E-14));
#20006=DIRECTION('center_axis',(-9.60574466455073E-15,-3.94255335449275E-30,
1.));
#20007=DIRECTION('ref_axis',(1.,-1.E-14,9.60574466455073E-15));
#20008=DIRECTION('',(1.E-14,1.,0.));
#20009=DIRECTION('center_axis',(-1.,1.E-14,-1.E-14));
#20010=DIRECTION('ref_axis',(-1.E-14,-1.,-2.64060752475192E-45));
#20011=DIRECTION('',(1.E-14,1.,0.));
#20012=DIRECTION('center_axis',(-1.E-14,0.,1.));
#20013=DIRECTION('ref_axis',(1.,-1.E-14,1.E-14));
#20014=DIRECTION('center_axis',(-9.60574466455073E-15,-3.94255335449275E-30,
1.));
#20015=DIRECTION('ref_axis',(1.,-1.E-14,9.60574466455073E-15));
#20016=DIRECTION('',(1.E-14,1.,0.));
#20017=DIRECTION('center_axis',(-1.,1.E-14,-1.E-14));
#20018=DIRECTION('ref_axis',(-1.E-14,-1.,-2.64060752475192E-45));
#20019=DIRECTION('',(1.E-14,1.,0.));
#20020=DIRECTION('center_axis',(-1.E-14,0.,1.));
#20021=DIRECTION('ref_axis',(1.,-1.E-14,1.E-14));
#20022=DIRECTION('center_axis',(-9.60574466455073E-15,-3.94255335449275E-30,
1.));
#20023=DIRECTION('ref_axis',(1.,-1.E-14,9.60574466455073E-15));
#20024=DIRECTION('',(1.E-14,1.,0.));
#20025=DIRECTION('center_axis',(-1.,1.E-14,-1.E-14));
#20026=DIRECTION('ref_axis',(-1.E-14,-1.,-2.64060752475192E-45));
#20027=DIRECTION('',(1.E-14,1.,0.));
#20028=DIRECTION('center_axis',(-1.E-14,0.,1.));
#20029=DIRECTION('ref_axis',(1.,-1.E-14,1.E-14));
#20030=DIRECTION('center_axis',(-9.60574466455073E-15,-3.94255335449275E-30,
1.));
#20031=DIRECTION('ref_axis',(1.,-1.E-14,9.60574466455073E-15));
#20032=DIRECTION('',(1.E-14,1.,0.));
#20033=DIRECTION('center_axis',(-1.,1.E-14,-1.E-14));
#20034=DIRECTION('ref_axis',(-1.E-14,-1.,-2.64060752475192E-45));
#20035=DIRECTION('',(1.E-14,1.,0.));
#20036=DIRECTION('center_axis',(-1.E-14,0.,1.));
#20037=DIRECTION('ref_axis',(1.,-1.E-14,1.E-14));
#20038=DIRECTION('center_axis',(-9.60574466455073E-15,-3.94255335449275E-30,
1.));
#20039=DIRECTION('ref_axis',(1.,-1.E-14,9.60574466455073E-15));
#20040=DIRECTION('',(1.E-14,1.,0.));
#20041=DIRECTION('center_axis',(-1.,1.E-14,-1.E-14));
#20042=DIRECTION('ref_axis',(-1.E-14,-1.,-2.64060752475192E-45));
#20043=DIRECTION('',(1.E-14,1.,0.));
#20044=DIRECTION('center_axis',(-1.E-14,0.,1.));
#20045=DIRECTION('ref_axis',(1.,-1.E-14,1.E-14));
#20046=DIRECTION('center_axis',(-9.60574466455072E-15,-3.94255335449275E-30,
1.));
#20047=DIRECTION('ref_axis',(1.,-1.E-14,9.60574466455072E-15));
#20048=DIRECTION('',(1.E-14,1.,0.));
#20049=DIRECTION('center_axis',(-1.,1.E-14,-1.E-14));
#20050=DIRECTION('ref_axis',(-1.E-14,-1.,-2.64060752475192E-45));
#20051=DIRECTION('',(1.E-14,1.,0.));
#20052=DIRECTION('center_axis',(-1.E-14,0.,1.));
#20053=DIRECTION('ref_axis',(1.,-1.E-14,1.E-14));
#20054=DIRECTION('center_axis',(-9.60574466455072E-15,-3.94255335449275E-30,
1.));
#20055=DIRECTION('ref_axis',(1.,-1.E-14,9.60574466455072E-15));
#20056=DIRECTION('',(1.E-14,1.,0.));
#20057=DIRECTION('center_axis',(-1.,1.E-14,-1.E-14));
#20058=DIRECTION('ref_axis',(-1.E-14,-1.,-2.64060752475192E-45));
#20059=DIRECTION('',(1.E-14,1.,0.));
#20060=DIRECTION('center_axis',(-1.E-14,0.,1.));
#20061=DIRECTION('ref_axis',(1.,-1.E-14,1.E-14));
#20062=DIRECTION('center_axis',(-9.60574466455072E-15,-3.94255335449275E-30,
1.));
#20063=DIRECTION('ref_axis',(1.,-1.E-14,9.60574466455072E-15));
#20064=DIRECTION('',(1.E-14,1.,0.));
#20065=DIRECTION('center_axis',(-1.,1.E-14,-1.E-14));
#20066=DIRECTION('ref_axis',(-1.E-14,-1.,-2.64060752475192E-45));
#20067=DIRECTION('',(1.E-14,1.,0.));
#20068=DIRECTION('center_axis',(-1.E-14,0.,1.));
#20069=DIRECTION('ref_axis',(1.,-1.E-14,1.E-14));
#20070=DIRECTION('center_axis',(-9.60574466455072E-15,-3.94255335449275E-30,
1.));
#20071=DIRECTION('ref_axis',(1.,-1.E-14,9.60574466455072E-15));
#20072=DIRECTION('',(1.E-14,1.,0.));
#20073=DIRECTION('center_axis',(-1.,1.E-14,-1.E-14));
#20074=DIRECTION('ref_axis',(-1.E-14,-1.,-2.64060752475192E-45));
#20075=DIRECTION('',(1.E-14,1.,0.));
#20076=DIRECTION('center_axis',(-1.E-14,0.,1.));
#20077=DIRECTION('ref_axis',(1.,-1.E-14,1.E-14));
#20078=DIRECTION('center_axis',(-9.60574466455072E-15,-3.94255335449275E-30,
1.));
#20079=DIRECTION('ref_axis',(1.,-1.E-14,9.60574466455072E-15));
#20080=DIRECTION('',(1.E-14,1.,0.));
#20081=DIRECTION('center_axis',(-1.,1.E-14,-1.E-14));
#20082=DIRECTION('ref_axis',(-1.E-14,-1.,-2.64060752475192E-45));
#20083=DIRECTION('',(1.E-14,1.,0.));
#20084=DIRECTION('center_axis',(-1.E-14,0.,1.));
#20085=DIRECTION('ref_axis',(1.,-1.E-14,1.E-14));
#20086=DIRECTION('center_axis',(-9.60574466455072E-15,-3.94255335449275E-30,
1.));
#20087=DIRECTION('ref_axis',(1.,-1.E-14,9.60574466455072E-15));
#20088=DIRECTION('',(1.E-14,1.,0.));
#20089=DIRECTION('center_axis',(-1.,1.E-14,-1.E-14));
#20090=DIRECTION('ref_axis',(-1.E-14,-1.,-2.64060752475192E-45));
#20091=DIRECTION('',(1.E-14,1.,0.));
#20092=DIRECTION('center_axis',(-1.E-14,0.,1.));
#20093=DIRECTION('ref_axis',(1.,-1.E-14,1.E-14));
#20094=DIRECTION('center_axis',(-9.60574466455072E-15,-3.94255335449275E-30,
1.));
#20095=DIRECTION('ref_axis',(1.,-1.E-14,9.60574466455072E-15));
#20096=DIRECTION('',(1.E-14,1.,0.));
#20097=DIRECTION('center_axis',(-1.,1.E-14,-1.E-14));
#20098=DIRECTION('ref_axis',(-1.E-14,-1.,-2.64060752475192E-45));
#20099=DIRECTION('',(1.E-14,1.,0.));
#20100=DIRECTION('center_axis',(-1.E-14,0.,1.));
#20101=DIRECTION('ref_axis',(1.,-1.E-14,1.E-14));
#20102=DIRECTION('center_axis',(-9.60574466455072E-15,-3.94255335449275E-30,
1.));
#20103=DIRECTION('ref_axis',(1.,-1.E-14,9.60574466455072E-15));
#20104=DIRECTION('',(1.E-14,1.,0.));
#20105=DIRECTION('center_axis',(-1.,1.E-14,-1.E-14));
#20106=DIRECTION('ref_axis',(-1.E-14,-1.,-2.64060752475192E-45));
#20107=DIRECTION('',(1.E-14,1.,0.));
#20108=DIRECTION('center_axis',(-1.E-14,0.,1.));
#20109=DIRECTION('ref_axis',(1.,-1.E-14,1.E-14));
#20110=DIRECTION('center_axis',(-9.60574466455072E-15,-3.94255335449275E-30,
1.));
#20111=DIRECTION('ref_axis',(1.,-1.E-14,9.60574466455072E-15));
#20112=DIRECTION('',(1.E-14,1.,0.));
#20113=DIRECTION('center_axis',(-1.,1.E-14,-1.E-14));
#20114=DIRECTION('ref_axis',(-1.E-14,-1.,-2.64060752475192E-45));
#20115=DIRECTION('',(1.E-14,1.,0.));
#20116=DIRECTION('center_axis',(-1.E-14,0.,1.));
#20117=DIRECTION('ref_axis',(1.,-1.E-14,1.E-14));
#20118=DIRECTION('center_axis',(-9.60574466455072E-15,-3.94255335449275E-30,
1.));
#20119=DIRECTION('ref_axis',(1.,-1.E-14,9.60574466455072E-15));
#20120=DIRECTION('',(1.E-14,1.,0.));
#20121=DIRECTION('center_axis',(-1.,1.E-14,-1.E-14));
#20122=DIRECTION('ref_axis',(-1.E-14,-1.,-2.64060752475192E-45));
#20123=DIRECTION('',(1.E-14,1.,0.));
#20124=DIRECTION('center_axis',(-1.E-14,0.,1.));
#20125=DIRECTION('ref_axis',(1.,-1.E-14,1.E-14));
#20126=DIRECTION('center_axis',(-9.60574466455072E-15,-3.94255335449275E-30,
1.));
#20127=DIRECTION('ref_axis',(1.,-1.E-14,9.60574466455072E-15));
#20128=DIRECTION('',(1.E-14,1.,0.));
#20129=DIRECTION('center_axis',(-1.,1.E-14,-1.E-14));
#20130=DIRECTION('ref_axis',(-1.E-14,-1.,-2.64060752475192E-45));
#20131=DIRECTION('',(1.E-14,1.,0.));
#20132=DIRECTION('center_axis',(-1.E-14,0.,1.));
#20133=DIRECTION('ref_axis',(1.,-1.E-14,1.E-14));
#20134=DIRECTION('center_axis',(-9.60574466455072E-15,-3.94255335449275E-30,
1.));
#20135=DIRECTION('ref_axis',(1.,-1.E-14,9.60574466455072E-15));
#20136=DIRECTION('',(1.E-14,1.,0.));
#20137=DIRECTION('center_axis',(-1.,1.E-14,-1.E-14));
#20138=DIRECTION('ref_axis',(-1.E-14,-1.,-2.64060752475192E-45));
#20139=DIRECTION('',(1.E-14,1.,0.));
#20140=DIRECTION('center_axis',(-1.E-14,0.,1.));
#20141=DIRECTION('ref_axis',(1.,-1.E-14,1.E-14));
#20142=DIRECTION('center_axis',(-9.60574466455072E-15,-3.94255335449275E-30,
1.));
#20143=DIRECTION('ref_axis',(1.,-1.E-14,9.60574466455072E-15));
#20144=DIRECTION('',(1.E-14,1.,0.));
#20145=DIRECTION('center_axis',(-1.,1.E-14,-1.E-14));
#20146=DIRECTION('ref_axis',(-1.E-14,-1.,-2.64060752475192E-45));
#20147=DIRECTION('',(1.E-14,1.,0.));
#20148=DIRECTION('center_axis',(-1.E-14,0.,1.));
#20149=DIRECTION('ref_axis',(1.,-1.E-14,1.E-14));
#20150=DIRECTION('center_axis',(-9.60574466455072E-15,-3.94255335449275E-30,
1.));
#20151=DIRECTION('ref_axis',(1.,-1.E-14,9.60574466455072E-15));
#20152=DIRECTION('',(1.E-14,1.,0.));
#20153=DIRECTION('center_axis',(-1.,1.E-14,-1.E-14));
#20154=DIRECTION('ref_axis',(-1.E-14,-1.,-2.64060752475192E-45));
#20155=DIRECTION('',(1.E-14,1.,0.));
#20156=DIRECTION('center_axis',(-1.E-14,0.,1.));
#20157=DIRECTION('ref_axis',(1.,-1.E-14,1.E-14));
#20158=DIRECTION('center_axis',(-9.60574466455072E-15,-3.94255335449275E-30,
1.));
#20159=DIRECTION('ref_axis',(1.,-1.E-14,9.60574466455072E-15));
#20160=DIRECTION('',(1.E-14,1.,0.));
#20161=DIRECTION('center_axis',(-1.,1.E-14,-1.E-14));
#20162=DIRECTION('ref_axis',(-1.E-14,-1.,-2.64060752475192E-45));
#20163=DIRECTION('',(1.E-14,1.,0.));
#20164=DIRECTION('center_axis',(-1.E-14,0.,1.));
#20165=DIRECTION('ref_axis',(1.,-1.E-14,1.E-14));
#20166=DIRECTION('center_axis',(1.,-1.E-14,0.));
#20167=DIRECTION('ref_axis',(1.E-14,1.,0.));
#24195=CARTESIAN_POINT('',(0.,0.,0.));
#24196=CARTESIAN_POINT('Origin',(-101.730458833643,31.763829283201,198.199999999999));
#24197=CARTESIAN_POINT('',(-85.6069914720345,31.7638292832008,210.499999999999));
#24198=CARTESIAN_POINT('',(-85.6069914720345,31.7638292832008,198.199999999999));
#24199=CARTESIAN_POINT('',(-85.6069914720345,31.7638292832008,194.611133062546));
#24200=CARTESIAN_POINT('',(18.2695411663569,31.7638292831998,210.5));
#24201=CARTESIAN_POINT('',(-101.730458833643,31.763829283201,210.499999999999));
#24202=CARTESIAN_POINT('',(18.269541166357,31.7638292831998,198.2));
#24203=CARTESIAN_POINT('',(18.269541166357,31.7638292831998,198.2));
#24204=CARTESIAN_POINT('',(-101.730458833643,31.763829283201,198.199999999999));
#24205=CARTESIAN_POINT('',(17.0195411663569,31.7638292831998,208.75));
#24206=CARTESIAN_POINT('Origin',(16.2695411663569,31.7638292831998,208.75));
#24207=CARTESIAN_POINT('',(13.0195411663569,31.7638292831999,208.75));
#24208=CARTESIAN_POINT('Origin',(12.2695411663569,31.7638292831999,208.75));
#24209=CARTESIAN_POINT('',(9.0195411663569,31.7638292831999,208.75));
#24210=CARTESIAN_POINT('Origin',(8.26954116635689,31.7638292831999,208.75));
#24211=CARTESIAN_POINT('',(5.01954116635689,31.7638292831999,208.75));
#24212=CARTESIAN_POINT('Origin',(4.26954116635689,31.7638292831999,208.75));
#24213=CARTESIAN_POINT('',(1.01954116635689,31.7638292832,208.75));
#24214=CARTESIAN_POINT('Origin',(0.269541166356885,31.7638292832,208.75));
#24215=CARTESIAN_POINT('',(-2.9804588336431,31.7638292832,208.75));
#24216=CARTESIAN_POINT('Origin',(-3.7304588336431,31.7638292832,208.75));
#24217=CARTESIAN_POINT('',(-6.9804588336431,31.7638292832001,208.75));
#24218=CARTESIAN_POINT('Origin',(-7.73045883364311,31.7638292832001,208.75));
#24219=CARTESIAN_POINT('',(-10.9804588336431,31.7638292832001,208.75));
#24220=CARTESIAN_POINT('Origin',(-11.7304588336431,31.7638292832001,208.75));
#24221=CARTESIAN_POINT('',(-14.9804588336431,31.7638292832001,208.75));
#24222=CARTESIAN_POINT('Origin',(-15.7304588336431,31.7638292832001,208.75));
#24223=CARTESIAN_POINT('',(-18.9804588336431,31.7638292832002,208.75));
#24224=CARTESIAN_POINT('Origin',(-19.7304588336431,31.7638292832002,208.75));
#24225=CARTESIAN_POINT('',(-22.9804588336431,31.7638292832002,208.75));
#24226=CARTESIAN_POINT('Origin',(-23.7304588336431,31.7638292832002,208.75));
#24227=CARTESIAN_POINT('',(-26.9804588336431,31.7638292832002,208.75));
#24228=CARTESIAN_POINT('Origin',(-27.7304588336431,31.7638292832003,208.75));
#24229=CARTESIAN_POINT('',(-30.9804588336431,31.7638292832003,208.75));
#24230=CARTESIAN_POINT('Origin',(-31.7304588336431,31.7638292832003,208.75));
#24231=CARTESIAN_POINT('',(-34.9804588336431,31.7638292832003,208.75));
#24232=CARTESIAN_POINT('Origin',(-35.7304588336431,31.7638292832003,208.75));
#24233=CARTESIAN_POINT('',(-38.9804588336431,31.7638292832004,208.75));
#24234=CARTESIAN_POINT('Origin',(-39.7304588336431,31.7638292832004,208.75));
#24235=CARTESIAN_POINT('',(-42.9804588336431,31.7638292832004,208.75));
#24236=CARTESIAN_POINT('Origin',(-43.7304588336431,31.7638292832004,208.75));
#24237=CARTESIAN_POINT('',(-46.9804588336431,31.7638292832005,208.75));
#24238=CARTESIAN_POINT('Origin',(-47.7304588336431,31.7638292832005,208.75));
#24239=CARTESIAN_POINT('',(-50.9804588336431,31.7638292832005,208.749999999999));
#24240=CARTESIAN_POINT('Origin',(-51.7304588336431,31.7638292832005,208.749999999999));
#24241=CARTESIAN_POINT('',(-54.9804588336431,31.7638292832005,208.749999999999));
#24242=CARTESIAN_POINT('Origin',(-55.7304588336431,31.7638292832005,208.749999999999));
#24243=CARTESIAN_POINT('',(-58.9804588336431,31.7638292832006,208.749999999999));
#24244=CARTESIAN_POINT('Origin',(-59.7304588336431,31.7638292832006,208.749999999999));
#24245=CARTESIAN_POINT('',(-62.9804588336431,31.7638292832006,208.749999999999));
#24246=CARTESIAN_POINT('Origin',(-63.7304588336431,31.7638292832006,208.749999999999));
#24247=CARTESIAN_POINT('',(-66.9804588336431,31.7638292832006,208.749999999999));
#24248=CARTESIAN_POINT('Origin',(-67.7304588336431,31.7638292832007,208.749999999999));
#24249=CARTESIAN_POINT('',(-70.9804588336431,31.7638292832007,208.749999999999));
#24250=CARTESIAN_POINT('Origin',(-71.7304588336431,31.7638292832007,208.749999999999));
#24251=CARTESIAN_POINT('',(-74.9804588336431,31.7638292832007,208.749999999999));
#24252=CARTESIAN_POINT('Origin',(-75.7304588336431,31.7638292832007,208.749999999999));
#24253=CARTESIAN_POINT('',(-78.9804588336431,31.7638292832008,208.749999999999));
#24254=CARTESIAN_POINT('Origin',(-79.7304588336431,31.7638292832008,208.749999999999));
#24255=CARTESIAN_POINT('',(-82.9804588336431,31.7638292832008,208.749999999999));
#24256=CARTESIAN_POINT('Origin',(-83.7304588336431,31.7638292832008,208.749999999999));
#24257=CARTESIAN_POINT('',(-84.830458833643,31.7638292832008,201.549999999999));
#24258=CARTESIAN_POINT('',(-82.630458833643,31.7638292832008,201.549999999999));
#24259=CARTESIAN_POINT('',(-101.730458833643,31.763829283201,201.549999999999));
#24260=CARTESIAN_POINT('',(-82.6304588336431,31.7638292832008,204.949999999999));
#24261=CARTESIAN_POINT('',(-82.630458833643,31.7638292832008,198.199999999999));
#24262=CARTESIAN_POINT('',(-84.8304588336431,31.7638292832008,204.949999999999));
#24263=CARTESIAN_POINT('',(-101.730458833643,31.763829283201,204.949999999999));
#24264=CARTESIAN_POINT('',(-84.830458833643,31.7638292832008,198.199999999999));
#24265=CARTESIAN_POINT('',(-80.830458833643,31.7638292832008,201.549999999999));
#24266=CARTESIAN_POINT('',(-78.630458833643,31.7638292832008,201.549999999999));
#24267=CARTESIAN_POINT('',(-101.730458833643,31.763829283201,201.549999999999));
#24268=CARTESIAN_POINT('',(-78.6304588336431,31.7638292832008,204.949999999999));
#24269=CARTESIAN_POINT('',(-78.630458833643,31.7638292832008,198.199999999999));
#24270=CARTESIAN_POINT('',(-80.8304588336431,31.7638292832008,204.949999999999));
#24271=CARTESIAN_POINT('',(-101.730458833643,31.763829283201,204.949999999999));
#24272=CARTESIAN_POINT('',(-80.830458833643,31.7638292832008,198.199999999999));
#24273=CARTESIAN_POINT('',(-76.830458833643,31.7638292832008,201.549999999999));
#24274=CARTESIAN_POINT('',(-74.630458833643,31.7638292832007,201.549999999999));
#24275=CARTESIAN_POINT('',(-101.730458833643,31.763829283201,201.549999999999));
#24276=CARTESIAN_POINT('',(-74.6304588336431,31.7638292832007,204.949999999999));
#24277=CARTESIAN_POINT('',(-74.630458833643,31.7638292832007,198.199999999999));
#24278=CARTESIAN_POINT('',(-76.8304588336431,31.7638292832008,204.949999999999));
#24279=CARTESIAN_POINT('',(-101.730458833643,31.763829283201,204.949999999999));
#24280=CARTESIAN_POINT('',(-76.830458833643,31.7638292832008,198.199999999999));
#24281=CARTESIAN_POINT('',(-72.830458833643,31.7638292832007,201.549999999999));
#24282=CARTESIAN_POINT('',(-70.630458833643,31.7638292832007,201.549999999999));
#24283=CARTESIAN_POINT('',(-101.730458833643,31.763829283201,201.549999999999));
#24284=CARTESIAN_POINT('',(-70.6304588336431,31.7638292832007,204.949999999999));
#24285=CARTESIAN_POINT('',(-70.630458833643,31.7638292832007,198.199999999999));
#24286=CARTESIAN_POINT('',(-72.8304588336431,31.7638292832007,204.949999999999));
#24287=CARTESIAN_POINT('',(-101.730458833643,31.763829283201,204.949999999999));
#24288=CARTESIAN_POINT('',(-72.830458833643,31.7638292832007,198.199999999999));
#24289=CARTESIAN_POINT('',(-68.830458833643,31.7638292832007,201.549999999999));
#24290=CARTESIAN_POINT('',(-66.630458833643,31.7638292832006,201.549999999999));
#24291=CARTESIAN_POINT('',(-101.730458833643,31.763829283201,201.549999999999));
#24292=CARTESIAN_POINT('',(-66.6304588336431,31.7638292832006,204.949999999999));
#24293=CARTESIAN_POINT('',(-66.630458833643,31.7638292832006,198.199999999999));
#24294=CARTESIAN_POINT('',(-68.8304588336431,31.7638292832007,204.949999999999));
#24295=CARTESIAN_POINT('',(-101.730458833643,31.763829283201,204.949999999999));
#24296=CARTESIAN_POINT('',(-68.830458833643,31.7638292832007,198.199999999999));
#24297=CARTESIAN_POINT('',(-64.830458833643,31.7638292832006,201.549999999999));
#24298=CARTESIAN_POINT('',(-62.630458833643,31.7638292832006,201.549999999999));
#24299=CARTESIAN_POINT('',(-101.730458833643,31.763829283201,201.549999999999));
#24300=CARTESIAN_POINT('',(-62.6304588336431,31.7638292832006,204.949999999999));
#24301=CARTESIAN_POINT('',(-62.630458833643,31.7638292832006,198.199999999999));
#24302=CARTESIAN_POINT('',(-64.8304588336431,31.7638292832006,204.949999999999));
#24303=CARTESIAN_POINT('',(-101.730458833643,31.763829283201,204.949999999999));
#24304=CARTESIAN_POINT('',(-64.830458833643,31.7638292832006,198.199999999999));
#24305=CARTESIAN_POINT('',(-60.830458833643,31.7638292832006,201.549999999999));
#24306=CARTESIAN_POINT('',(-58.630458833643,31.7638292832006,201.549999999999));
#24307=CARTESIAN_POINT('',(-101.730458833643,31.763829283201,201.549999999999));
#24308=CARTESIAN_POINT('',(-58.6304588336431,31.7638292832006,204.949999999999));
#24309=CARTESIAN_POINT('',(-58.630458833643,31.7638292832006,198.199999999999));
#24310=CARTESIAN_POINT('',(-60.8304588336431,31.7638292832006,204.949999999999));
#24311=CARTESIAN_POINT('',(-101.730458833643,31.763829283201,204.949999999999));
#24312=CARTESIAN_POINT('',(-60.830458833643,31.7638292832006,198.199999999999));
#24313=CARTESIAN_POINT('',(-56.830458833643,31.7638292832006,201.549999999999));
#24314=CARTESIAN_POINT('',(-54.630458833643,31.7638292832005,201.549999999999));
#24315=CARTESIAN_POINT('',(-101.730458833643,31.763829283201,201.549999999999));
#24316=CARTESIAN_POINT('',(-54.6304588336431,31.7638292832005,204.949999999999));
#24317=CARTESIAN_POINT('',(-54.630458833643,31.7638292832005,198.199999999999));
#24318=CARTESIAN_POINT('',(-56.8304588336431,31.7638292832006,204.949999999999));
#24319=CARTESIAN_POINT('',(-101.730458833643,31.763829283201,204.949999999999));
#24320=CARTESIAN_POINT('',(-56.830458833643,31.7638292832006,198.199999999999));
#24321=CARTESIAN_POINT('',(-52.830458833643,31.7638292832005,201.549999999999));
#24322=CARTESIAN_POINT('',(-50.630458833643,31.7638292832005,201.549999999999));
#24323=CARTESIAN_POINT('',(-101.730458833643,31.763829283201,201.549999999999));
#24324=CARTESIAN_POINT('',(-50.6304588336431,31.7638292832005,204.95));
#24325=CARTESIAN_POINT('',(-50.630458833643,31.7638292832005,198.2));
#24326=CARTESIAN_POINT('',(-52.8304588336431,31.7638292832005,204.949999999999));
#24327=CARTESIAN_POINT('',(-101.730458833643,31.763829283201,204.949999999999));
#24328=CARTESIAN_POINT('',(-52.830458833643,31.7638292832005,198.2));
#24329=CARTESIAN_POINT('',(-48.830458833643,31.7638292832005,201.549999999999));
#24330=CARTESIAN_POINT('',(-46.630458833643,31.7638292832005,201.55));
#24331=CARTESIAN_POINT('',(-101.730458833643,31.763829283201,201.549999999999));
#24332=CARTESIAN_POINT('',(-46.6304588336431,31.7638292832005,204.95));
#24333=CARTESIAN_POINT('',(-46.630458833643,31.7638292832005,198.2));
#24334=CARTESIAN_POINT('',(-48.8304588336431,31.7638292832005,204.95));
#24335=CARTESIAN_POINT('',(-101.730458833643,31.763829283201,204.949999999999));
#24336=CARTESIAN_POINT('',(-48.830458833643,31.7638292832005,198.2));
#24337=CARTESIAN_POINT('',(-44.830458833643,31.7638292832004,201.55));
#24338=CARTESIAN_POINT('',(-42.630458833643,31.7638292832004,201.55));
#24339=CARTESIAN_POINT('',(-101.730458833643,31.763829283201,201.549999999999));
#24340=CARTESIAN_POINT('',(-42.6304588336431,31.7638292832004,204.95));
#24341=CARTESIAN_POINT('',(-42.630458833643,31.7638292832004,198.2));
#24342=CARTESIAN_POINT('',(-44.8304588336431,31.7638292832004,204.95));
#24343=CARTESIAN_POINT('',(-101.730458833643,31.763829283201,204.949999999999));
#24344=CARTESIAN_POINT('',(-44.830458833643,31.7638292832004,198.2));
#24345=CARTESIAN_POINT('',(-40.830458833643,31.7638292832004,201.55));
#24346=CARTESIAN_POINT('',(-38.630458833643,31.7638292832004,201.55));
#24347=CARTESIAN_POINT('',(-101.730458833643,31.763829283201,201.549999999999));
#24348=CARTESIAN_POINT('',(-38.6304588336431,31.7638292832004,204.95));
#24349=CARTESIAN_POINT('',(-38.630458833643,31.7638292832004,198.2));
#24350=CARTESIAN_POINT('',(-40.8304588336431,31.7638292832004,204.95));
#24351=CARTESIAN_POINT('',(-101.730458833643,31.763829283201,204.949999999999));
#24352=CARTESIAN_POINT('',(-40.830458833643,31.7638292832004,198.2));
#24353=CARTESIAN_POINT('',(-36.830458833643,31.7638292832003,201.55));
#24354=CARTESIAN_POINT('',(-34.630458833643,31.7638292832003,201.55));
#24355=CARTESIAN_POINT('',(-101.730458833643,31.763829283201,201.549999999999));
#24356=CARTESIAN_POINT('',(-34.6304588336431,31.7638292832003,204.95));
#24357=CARTESIAN_POINT('',(-34.630458833643,31.7638292832003,198.2));
#24358=CARTESIAN_POINT('',(-36.8304588336431,31.7638292832003,204.95));
#24359=CARTESIAN_POINT('',(-101.730458833643,31.763829283201,204.949999999999));
#24360=CARTESIAN_POINT('',(-36.830458833643,31.7638292832003,198.2));
#24361=CARTESIAN_POINT('',(-32.830458833643,31.7638292832003,201.55));
#24362=CARTESIAN_POINT('',(-30.630458833643,31.7638292832003,201.55));
#24363=CARTESIAN_POINT('',(-101.730458833643,31.763829283201,201.549999999999));
#24364=CARTESIAN_POINT('',(-30.6304588336431,31.7638292832003,204.95));
#24365=CARTESIAN_POINT('',(-30.630458833643,31.7638292832003,198.2));
#24366=CARTESIAN_POINT('',(-32.8304588336431,31.7638292832003,204.95));
#24367=CARTESIAN_POINT('',(-101.730458833643,31.763829283201,204.949999999999));
#24368=CARTESIAN_POINT('',(-32.830458833643,31.7638292832003,198.2));
#24369=CARTESIAN_POINT('',(-28.830458833643,31.7638292832003,201.55));
#24370=CARTESIAN_POINT('',(-26.630458833643,31.7638292832003,201.55));
#24371=CARTESIAN_POINT('',(-101.730458833643,31.763829283201,201.549999999999));
#24372=CARTESIAN_POINT('',(-26.6304588336431,31.7638292832003,204.95));
#24373=CARTESIAN_POINT('',(-26.630458833643,31.7638292832003,198.2));
#24374=CARTESIAN_POINT('',(-28.8304588336431,31.7638292832003,204.95));
#24375=CARTESIAN_POINT('',(-101.730458833643,31.763829283201,204.949999999999));
#24376=CARTESIAN_POINT('',(-28.830458833643,31.7638292832003,198.2));
#24377=CARTESIAN_POINT('',(-24.830458833643,31.7638292832002,201.55));
#24378=CARTESIAN_POINT('',(-22.630458833643,31.7638292832002,201.55));
#24379=CARTESIAN_POINT('',(-101.730458833643,31.763829283201,201.549999999999));
#24380=CARTESIAN_POINT('',(-22.6304588336431,31.7638292832002,204.95));
#24381=CARTESIAN_POINT('',(-22.630458833643,31.7638292832002,198.2));
#24382=CARTESIAN_POINT('',(-24.8304588336431,31.7638292832002,204.95));
#24383=CARTESIAN_POINT('',(-101.730458833643,31.763829283201,204.949999999999));
#24384=CARTESIAN_POINT('',(-24.830458833643,31.7638292832002,198.2));
#24385=CARTESIAN_POINT('',(-20.830458833643,31.7638292832002,201.55));
#24386=CARTESIAN_POINT('',(-18.630458833643,31.7638292832002,201.55));
#24387=CARTESIAN_POINT('',(-101.730458833643,31.763829283201,201.549999999999));
#24388=CARTESIAN_POINT('',(-18.6304588336431,31.7638292832002,204.95));
#24389=CARTESIAN_POINT('',(-18.630458833643,31.7638292832002,198.2));
#24390=CARTESIAN_POINT('',(-20.8304588336431,31.7638292832002,204.95));
#24391=CARTESIAN_POINT('',(-101.730458833643,31.763829283201,204.949999999999));
#24392=CARTESIAN_POINT('',(-20.830458833643,31.7638292832002,198.2));
#24393=CARTESIAN_POINT('',(-16.830458833643,31.7638292832002,201.55));
#24394=CARTESIAN_POINT('',(-14.630458833643,31.7638292832001,201.55));
#24395=CARTESIAN_POINT('',(-101.730458833643,31.763829283201,201.549999999999));
#24396=CARTESIAN_POINT('',(-14.6304588336431,31.7638292832001,204.95));
#24397=CARTESIAN_POINT('',(-14.630458833643,31.7638292832001,198.2));
#24398=CARTESIAN_POINT('',(-16.8304588336431,31.7638292832002,204.95));
#24399=CARTESIAN_POINT('',(-101.730458833643,31.763829283201,204.949999999999));
#24400=CARTESIAN_POINT('',(-16.830458833643,31.7638292832002,198.2));
#24401=CARTESIAN_POINT('',(-12.830458833643,31.7638292832001,201.55));
#24402=CARTESIAN_POINT('',(-10.630458833643,31.7638292832001,201.55));
#24403=CARTESIAN_POINT('',(-101.730458833643,31.763829283201,201.549999999999));
#24404=CARTESIAN_POINT('',(-10.6304588336431,31.7638292832001,204.95));
#24405=CARTESIAN_POINT('',(-10.630458833643,31.7638292832001,198.2));
#24406=CARTESIAN_POINT('',(-12.8304588336431,31.7638292832001,204.95));
#24407=CARTESIAN_POINT('',(-101.730458833643,31.763829283201,204.949999999999));
#24408=CARTESIAN_POINT('',(-12.830458833643,31.7638292832001,198.2));
#24409=CARTESIAN_POINT('',(-8.83045883364303,31.7638292832001,201.55));
#24410=CARTESIAN_POINT('',(-6.63045883364302,31.7638292832,201.55));
#24411=CARTESIAN_POINT('',(-101.730458833643,31.763829283201,201.549999999999));
#24412=CARTESIAN_POINT('',(-6.63045883364306,31.7638292832,204.95));
#24413=CARTESIAN_POINT('',(-6.63045883364299,31.7638292832,198.2));
#24414=CARTESIAN_POINT('',(-8.83045883364307,31.7638292832001,204.95));
#24415=CARTESIAN_POINT('',(-101.730458833643,31.763829283201,204.949999999999));
#24416=CARTESIAN_POINT('',(-8.830458833643,31.7638292832001,198.2));
#24417=CARTESIAN_POINT('',(-4.83045883364302,31.7638292832,201.55));
#24418=CARTESIAN_POINT('',(-2.63045883364303,31.7638292832,201.55));
#24419=CARTESIAN_POINT('',(-101.730458833643,31.763829283201,201.549999999999));
#24420=CARTESIAN_POINT('',(-2.63045883364307,31.7638292832,204.95));
#24421=CARTESIAN_POINT('',(-2.630458833643,31.7638292832,198.2));
#24422=CARTESIAN_POINT('',(-4.83045883364307,31.7638292832,204.95));
#24423=CARTESIAN_POINT('',(-101.730458833643,31.763829283201,204.949999999999));
#24424=CARTESIAN_POINT('',(-4.830458833643,31.7638292832,198.2));
#24425=CARTESIAN_POINT('',(-0.830458833643022,31.7638292832,201.55));
#24426=CARTESIAN_POINT('',(1.36954116635697,31.7638292832,201.55));
#24427=CARTESIAN_POINT('',(-101.730458833643,31.763829283201,201.549999999999));
#24428=CARTESIAN_POINT('',(1.36954116635693,31.7638292832,204.95));
#24429=CARTESIAN_POINT('',(1.369541166357,31.7638292832,198.2));
#24430=CARTESIAN_POINT('',(-0.830458833643063,31.7638292832,204.95));
#24431=CARTESIAN_POINT('',(-101.730458833643,31.763829283201,204.949999999999));
#24432=CARTESIAN_POINT('',(-0.830458833642994,31.7638292832,198.2));
#24433=CARTESIAN_POINT('',(3.16954116635697,31.7638292832,201.55));
#24434=CARTESIAN_POINT('',(5.36954116635698,31.7638292831999,201.55));
#24435=CARTESIAN_POINT('',(-101.730458833643,31.763829283201,201.549999999999));
#24436=CARTESIAN_POINT('',(5.36954116635693,31.7638292831999,204.95));
#24437=CARTESIAN_POINT('',(5.369541166357,31.7638292831999,198.2));
#24438=CARTESIAN_POINT('',(3.16954116635693,31.7638292832,204.95));
#24439=CARTESIAN_POINT('',(-101.730458833643,31.763829283201,204.949999999999));
#24440=CARTESIAN_POINT('',(3.169541166357,31.7638292832,198.2));
#24441=CARTESIAN_POINT('',(7.16954116635697,31.7638292831999,201.55));
#24442=CARTESIAN_POINT('',(9.36954116635698,31.7638292831999,201.55));
#24443=CARTESIAN_POINT('',(-101.730458833643,31.763829283201,201.549999999999));
#24444=CARTESIAN_POINT('',(9.36954116635694,31.7638292831999,204.95));
#24445=CARTESIAN_POINT('',(9.36954116635701,31.7638292831999,198.2));
#24446=CARTESIAN_POINT('',(7.16954116635693,31.7638292831999,204.95));
#24447=CARTESIAN_POINT('',(-101.730458833643,31.763829283201,204.949999999999));
#24448=CARTESIAN_POINT('',(7.169541166357,31.7638292831999,198.2));
#24449=CARTESIAN_POINT('',(11.169541166357,31.7638292831999,201.55));
#24450=CARTESIAN_POINT('',(13.369541166357,31.7638292831998,201.55));
#24451=CARTESIAN_POINT('',(-101.730458833643,31.763829283201,201.549999999999));
#24452=CARTESIAN_POINT('',(13.3695411663569,31.7638292831998,204.95));
#24453=CARTESIAN_POINT('',(13.369541166357,31.7638292831998,198.2));
#24454=CARTESIAN_POINT('',(11.1695411663569,31.7638292831999,204.95));
#24455=CARTESIAN_POINT('',(-101.730458833643,31.763829283201,204.949999999999));
#24456=CARTESIAN_POINT('',(11.169541166357,31.7638292831999,198.2));
#24457=CARTESIAN_POINT('',(15.169541166357,31.7638292831998,201.55));
#24458=CARTESIAN_POINT('',(17.369541166357,31.7638292831998,201.55));
#24459=CARTESIAN_POINT('',(-101.730458833643,31.763829283201,201.549999999999));
#24460=CARTESIAN_POINT('',(17.3695411663569,31.7638292831998,204.95));
#24461=CARTESIAN_POINT('',(17.369541166357,31.7638292831998,198.2));
#24462=CARTESIAN_POINT('',(15.1695411663569,31.7638292831998,204.95));
#24463=CARTESIAN_POINT('',(-101.730458833643,31.763829283201,204.949999999999));
#24464=CARTESIAN_POINT('',(15.169541166357,31.7638292831998,198.2));
#24465=CARTESIAN_POINT('Origin',(-101.730458833643,31.263829283201,198.199999999999));
#24466=CARTESIAN_POINT('',(-85.6069914720345,31.2638292831998,198.199999999999));
#24467=CARTESIAN_POINT('',(-85.6069914720345,31.2638292832008,210.5));
#24468=CARTESIAN_POINT('',(-85.6069914720345,31.2638292832008,198.199999999999));
#24469=CARTESIAN_POINT('',(18.269541166357,31.2638292831998,198.2));
#24470=CARTESIAN_POINT('',(-101.730458833643,31.263829283201,198.199999999999));
#24471=CARTESIAN_POINT('',(18.2695411663569,31.2638292831998,210.5));
#24472=CARTESIAN_POINT('',(18.269541166357,31.2638292831998,198.2));
#24473=CARTESIAN_POINT('',(-101.730458833643,31.263829283201,210.499999999999));
#24474=CARTESIAN_POINT('',(15.169541166357,31.2638292831998,201.55));
#24475=CARTESIAN_POINT('',(17.369541166357,31.2638292831998,201.55));
#24476=CARTESIAN_POINT('',(-101.730458833643,31.263829283201,201.549999999999));
#24477=CARTESIAN_POINT('',(15.1695411663569,31.2638292831998,204.95));
#24478=CARTESIAN_POINT('',(15.169541166357,31.2638292831998,198.2));
#24479=CARTESIAN_POINT('',(17.3695411663569,31.2638292831998,204.95));
#24480=CARTESIAN_POINT('',(-101.730458833643,31.263829283201,204.949999999999));
#24481=CARTESIAN_POINT('',(17.369541166357,31.2638292831998,198.2));
#24482=CARTESIAN_POINT('',(11.169541166357,31.2638292831999,201.55));
#24483=CARTESIAN_POINT('',(13.369541166357,31.2638292831998,201.55));
#24484=CARTESIAN_POINT('',(-101.730458833643,31.263829283201,201.549999999999));
#24485=CARTESIAN_POINT('',(11.1695411663569,31.2638292831999,204.95));
#24486=CARTESIAN_POINT('',(11.169541166357,31.2638292831999,198.2));
#24487=CARTESIAN_POINT('',(13.3695411663569,31.2638292831998,204.95));
#24488=CARTESIAN_POINT('',(-101.730458833643,31.263829283201,204.949999999999));
#24489=CARTESIAN_POINT('',(13.369541166357,31.2638292831998,198.2));
#24490=CARTESIAN_POINT('',(7.16954116635697,31.2638292831999,201.55));
#24491=CARTESIAN_POINT('',(9.36954116635698,31.2638292831999,201.55));
#24492=CARTESIAN_POINT('',(-101.730458833643,31.263829283201,201.549999999999));
#24493=CARTESIAN_POINT('',(7.16954116635693,31.2638292831999,204.95));
#24494=CARTESIAN_POINT('',(7.169541166357,31.2638292831999,198.2));
#24495=CARTESIAN_POINT('',(9.36954116635694,31.2638292831999,204.95));
#24496=CARTESIAN_POINT('',(-101.730458833643,31.263829283201,204.949999999999));
#24497=CARTESIAN_POINT('',(9.36954116635701,31.2638292831999,198.2));
#24498=CARTESIAN_POINT('',(3.16954116635697,31.2638292832,201.55));
#24499=CARTESIAN_POINT('',(5.36954116635698,31.2638292831999,201.55));
#24500=CARTESIAN_POINT('',(-101.730458833643,31.263829283201,201.549999999999));
#24501=CARTESIAN_POINT('',(3.16954116635693,31.2638292832,204.95));
#24502=CARTESIAN_POINT('',(3.169541166357,31.2638292832,198.2));
#24503=CARTESIAN_POINT('',(5.36954116635693,31.2638292831999,204.95));
#24504=CARTESIAN_POINT('',(-101.730458833643,31.263829283201,204.949999999999));
#24505=CARTESIAN_POINT('',(5.369541166357,31.2638292831999,198.2));
#24506=CARTESIAN_POINT('',(-0.830458833643022,31.2638292832,201.55));
#24507=CARTESIAN_POINT('',(1.36954116635697,31.2638292832,201.55));
#24508=CARTESIAN_POINT('',(-101.730458833643,31.263829283201,201.549999999999));
#24509=CARTESIAN_POINT('',(-0.830458833643063,31.2638292832,204.95));
#24510=CARTESIAN_POINT('',(-0.830458833642994,31.2638292832,198.2));
#24511=CARTESIAN_POINT('',(1.36954116635693,31.2638292832,204.95));
#24512=CARTESIAN_POINT('',(-101.730458833643,31.263829283201,204.949999999999));
#24513=CARTESIAN_POINT('',(1.369541166357,31.2638292832,198.2));
#24514=CARTESIAN_POINT('',(-4.83045883364302,31.2638292832,201.55));
#24515=CARTESIAN_POINT('',(-2.63045883364303,31.2638292832,201.55));
#24516=CARTESIAN_POINT('',(-101.730458833643,31.263829283201,201.549999999999));
#24517=CARTESIAN_POINT('',(-4.83045883364307,31.2638292832,204.95));
#24518=CARTESIAN_POINT('',(-4.830458833643,31.2638292832,198.2));
#24519=CARTESIAN_POINT('',(-2.63045883364307,31.2638292832,204.95));
#24520=CARTESIAN_POINT('',(-101.730458833643,31.263829283201,204.949999999999));
#24521=CARTESIAN_POINT('',(-2.630458833643,31.2638292832,198.2));
#24522=CARTESIAN_POINT('',(-8.83045883364303,31.2638292832001,201.55));
#24523=CARTESIAN_POINT('',(-6.63045883364302,31.2638292832,201.55));
#24524=CARTESIAN_POINT('',(-101.730458833643,31.263829283201,201.549999999999));
#24525=CARTESIAN_POINT('',(-8.83045883364307,31.2638292832001,204.95));
#24526=CARTESIAN_POINT('',(-8.830458833643,31.2638292832001,198.2));
#24527=CARTESIAN_POINT('',(-6.63045883364306,31.2638292832,204.95));
#24528=CARTESIAN_POINT('',(-101.730458833643,31.263829283201,204.949999999999));
#24529=CARTESIAN_POINT('',(-6.63045883364299,31.2638292832,198.2));
#24530=CARTESIAN_POINT('',(-12.830458833643,31.2638292832001,201.55));
#24531=CARTESIAN_POINT('',(-10.630458833643,31.2638292832001,201.55));
#24532=CARTESIAN_POINT('',(-101.730458833643,31.263829283201,201.549999999999));
#24533=CARTESIAN_POINT('',(-12.8304588336431,31.2638292832001,204.95));
#24534=CARTESIAN_POINT('',(-12.830458833643,31.2638292832001,198.2));
#24535=CARTESIAN_POINT('',(-10.6304588336431,31.2638292832001,204.95));
#24536=CARTESIAN_POINT('',(-101.730458833643,31.263829283201,204.949999999999));
#24537=CARTESIAN_POINT('',(-10.630458833643,31.2638292832001,198.2));
#24538=CARTESIAN_POINT('',(-16.830458833643,31.2638292832002,201.55));
#24539=CARTESIAN_POINT('',(-14.630458833643,31.2638292832001,201.55));
#24540=CARTESIAN_POINT('',(-101.730458833643,31.263829283201,201.549999999999));
#24541=CARTESIAN_POINT('',(-16.8304588336431,31.2638292832002,204.95));
#24542=CARTESIAN_POINT('',(-16.830458833643,31.2638292832002,198.2));
#24543=CARTESIAN_POINT('',(-14.6304588336431,31.2638292832001,204.95));
#24544=CARTESIAN_POINT('',(-101.730458833643,31.263829283201,204.949999999999));
#24545=CARTESIAN_POINT('',(-14.630458833643,31.2638292832001,198.2));
#24546=CARTESIAN_POINT('',(-20.830458833643,31.2638292832002,201.55));
#24547=CARTESIAN_POINT('',(-18.630458833643,31.2638292832002,201.55));
#24548=CARTESIAN_POINT('',(-101.730458833643,31.263829283201,201.549999999999));
#24549=CARTESIAN_POINT('',(-20.8304588336431,31.2638292832002,204.95));
#24550=CARTESIAN_POINT('',(-20.830458833643,31.2638292832002,198.2));
#24551=CARTESIAN_POINT('',(-18.6304588336431,31.2638292832002,204.95));
#24552=CARTESIAN_POINT('',(-101.730458833643,31.263829283201,204.949999999999));
#24553=CARTESIAN_POINT('',(-18.630458833643,31.2638292832002,198.2));
#24554=CARTESIAN_POINT('',(-24.830458833643,31.2638292832002,201.55));
#24555=CARTESIAN_POINT('',(-22.630458833643,31.2638292832002,201.55));
#24556=CARTESIAN_POINT('',(-101.730458833643,31.263829283201,201.549999999999));
#24557=CARTESIAN_POINT('',(-24.8304588336431,31.2638292832002,204.95));
#24558=CARTESIAN_POINT('',(-24.830458833643,31.2638292832002,198.2));
#24559=CARTESIAN_POINT('',(-22.6304588336431,31.2638292832002,204.95));
#24560=CARTESIAN_POINT('',(-101.730458833643,31.263829283201,204.949999999999));
#24561=CARTESIAN_POINT('',(-22.630458833643,31.2638292832002,198.2));
#24562=CARTESIAN_POINT('',(-28.830458833643,31.2638292832003,201.55));
#24563=CARTESIAN_POINT('',(-26.630458833643,31.2638292832002,201.55));
#24564=CARTESIAN_POINT('',(-101.730458833643,31.263829283201,201.549999999999));
#24565=CARTESIAN_POINT('',(-28.8304588336431,31.2638292832003,204.95));
#24566=CARTESIAN_POINT('',(-28.830458833643,31.2638292832003,198.2));
#24567=CARTESIAN_POINT('',(-26.6304588336431,31.2638292832002,204.95));
#24568=CARTESIAN_POINT('',(-101.730458833643,31.263829283201,204.949999999999));
#24569=CARTESIAN_POINT('',(-26.630458833643,31.2638292832002,198.2));
#24570=CARTESIAN_POINT('',(-32.830458833643,31.2638292832003,201.55));
#24571=CARTESIAN_POINT('',(-30.630458833643,31.2638292832003,201.55));
#24572=CARTESIAN_POINT('',(-101.730458833643,31.263829283201,201.549999999999));
#24573=CARTESIAN_POINT('',(-32.8304588336431,31.2638292832003,204.95));
#24574=CARTESIAN_POINT('',(-32.830458833643,31.2638292832003,198.2));
#24575=CARTESIAN_POINT('',(-30.6304588336431,31.2638292832003,204.95));
#24576=CARTESIAN_POINT('',(-101.730458833643,31.263829283201,204.949999999999));
#24577=CARTESIAN_POINT('',(-30.630458833643,31.2638292832003,198.2));
#24578=CARTESIAN_POINT('',(-36.830458833643,31.2638292832004,201.55));
#24579=CARTESIAN_POINT('',(-34.630458833643,31.2638292832003,201.55));
#24580=CARTESIAN_POINT('',(-101.730458833643,31.263829283201,201.549999999999));
#24581=CARTESIAN_POINT('',(-36.8304588336431,31.2638292832004,204.95));
#24582=CARTESIAN_POINT('',(-36.830458833643,31.2638292832004,198.2));
#24583=CARTESIAN_POINT('',(-34.6304588336431,31.2638292832003,204.95));
#24584=CARTESIAN_POINT('',(-101.730458833643,31.263829283201,204.949999999999));
#24585=CARTESIAN_POINT('',(-34.630458833643,31.2638292832003,198.2));
#24586=CARTESIAN_POINT('',(-40.830458833643,31.2638292832004,201.55));
#24587=CARTESIAN_POINT('',(-38.630458833643,31.2638292832004,201.55));
#24588=CARTESIAN_POINT('',(-101.730458833643,31.263829283201,201.549999999999));
#24589=CARTESIAN_POINT('',(-40.8304588336431,31.2638292832004,204.95));
#24590=CARTESIAN_POINT('',(-40.830458833643,31.2638292832004,198.2));
#24591=CARTESIAN_POINT('',(-38.6304588336431,31.2638292832004,204.95));
#24592=CARTESIAN_POINT('',(-101.730458833643,31.263829283201,204.949999999999));
#24593=CARTESIAN_POINT('',(-38.630458833643,31.2638292832004,198.2));
#24594=CARTESIAN_POINT('',(-44.830458833643,31.2638292832004,201.55));
#24595=CARTESIAN_POINT('',(-42.630458833643,31.2638292832004,201.55));
#24596=CARTESIAN_POINT('',(-101.730458833643,31.263829283201,201.549999999999));
#24597=CARTESIAN_POINT('',(-44.8304588336431,31.2638292832004,204.95));
#24598=CARTESIAN_POINT('',(-44.830458833643,31.2638292832004,198.2));
#24599=CARTESIAN_POINT('',(-42.6304588336431,31.2638292832004,204.95));
#24600=CARTESIAN_POINT('',(-101.730458833643,31.263829283201,204.949999999999));
#24601=CARTESIAN_POINT('',(-42.630458833643,31.2638292832004,198.2));
#24602=CARTESIAN_POINT('',(-48.830458833643,31.2638292832005,201.549999999999));
#24603=CARTESIAN_POINT('',(-46.630458833643,31.2638292832004,201.55));
#24604=CARTESIAN_POINT('',(-101.730458833643,31.263829283201,201.549999999999));
#24605=CARTESIAN_POINT('',(-48.8304588336431,31.2638292832005,204.95));
#24606=CARTESIAN_POINT('',(-48.830458833643,31.2638292832005,198.2));
#24607=CARTESIAN_POINT('',(-46.6304588336431,31.2638292832004,204.95));
#24608=CARTESIAN_POINT('',(-101.730458833643,31.263829283201,204.949999999999));
#24609=CARTESIAN_POINT('',(-46.630458833643,31.2638292832004,198.2));
#24610=CARTESIAN_POINT('',(-52.830458833643,31.2638292832005,201.549999999999));
#24611=CARTESIAN_POINT('',(-50.630458833643,31.2638292832005,201.549999999999));
#24612=CARTESIAN_POINT('',(-101.730458833643,31.263829283201,201.549999999999));
#24613=CARTESIAN_POINT('',(-52.8304588336431,31.2638292832005,204.949999999999));
#24614=CARTESIAN_POINT('',(-52.830458833643,31.2638292832005,198.2));
#24615=CARTESIAN_POINT('',(-50.6304588336431,31.2638292832005,204.95));
#24616=CARTESIAN_POINT('',(-101.730458833643,31.263829283201,204.949999999999));
#24617=CARTESIAN_POINT('',(-50.630458833643,31.2638292832005,198.2));
#24618=CARTESIAN_POINT('',(-56.830458833643,31.2638292832006,201.549999999999));
#24619=CARTESIAN_POINT('',(-54.630458833643,31.2638292832005,201.549999999999));
#24620=CARTESIAN_POINT('',(-101.730458833643,31.263829283201,201.549999999999));
#24621=CARTESIAN_POINT('',(-56.8304588336431,31.2638292832006,204.949999999999));
#24622=CARTESIAN_POINT('',(-56.830458833643,31.2638292832006,198.199999999999));
#24623=CARTESIAN_POINT('',(-54.6304588336431,31.2638292832005,204.949999999999));
#24624=CARTESIAN_POINT('',(-101.730458833643,31.263829283201,204.949999999999));
#24625=CARTESIAN_POINT('',(-54.630458833643,31.2638292832005,198.199999999999));
#24626=CARTESIAN_POINT('',(-60.830458833643,31.2638292832006,201.549999999999));
#24627=CARTESIAN_POINT('',(-58.630458833643,31.2638292832006,201.549999999999));
#24628=CARTESIAN_POINT('',(-101.730458833643,31.263829283201,201.549999999999));
#24629=CARTESIAN_POINT('',(-60.8304588336431,31.2638292832006,204.949999999999));
#24630=CARTESIAN_POINT('',(-60.830458833643,31.2638292832006,198.199999999999));
#24631=CARTESIAN_POINT('',(-58.6304588336431,31.2638292832006,204.949999999999));
#24632=CARTESIAN_POINT('',(-101.730458833643,31.263829283201,204.949999999999));
#24633=CARTESIAN_POINT('',(-58.630458833643,31.2638292832006,198.199999999999));
#24634=CARTESIAN_POINT('',(-64.830458833643,31.2638292832006,201.549999999999));
#24635=CARTESIAN_POINT('',(-62.6304588336431,31.2638292832006,201.549999999999));
#24636=CARTESIAN_POINT('',(-101.730458833643,31.263829283201,201.549999999999));
#24637=CARTESIAN_POINT('',(-64.8304588336431,31.2638292832006,204.949999999999));
#24638=CARTESIAN_POINT('',(-64.830458833643,31.2638292832006,198.199999999999));
#24639=CARTESIAN_POINT('',(-62.6304588336431,31.2638292832006,204.949999999999));
#24640=CARTESIAN_POINT('',(-101.730458833643,31.263829283201,204.949999999999));
#24641=CARTESIAN_POINT('',(-62.630458833643,31.2638292832006,198.199999999999));
#24642=CARTESIAN_POINT('',(-68.830458833643,31.2638292832007,201.549999999999));
#24643=CARTESIAN_POINT('',(-66.630458833643,31.2638292832006,201.549999999999));
#24644=CARTESIAN_POINT('',(-101.730458833643,31.263829283201,201.549999999999));
#24645=CARTESIAN_POINT('',(-68.8304588336431,31.2638292832007,204.949999999999));
#24646=CARTESIAN_POINT('',(-68.830458833643,31.2638292832007,198.199999999999));
#24647=CARTESIAN_POINT('',(-66.6304588336431,31.2638292832006,204.949999999999));
#24648=CARTESIAN_POINT('',(-101.730458833643,31.263829283201,204.949999999999));
#24649=CARTESIAN_POINT('',(-66.630458833643,31.2638292832006,198.199999999999));
#24650=CARTESIAN_POINT('',(-72.830458833643,31.2638292832007,201.549999999999));
#24651=CARTESIAN_POINT('',(-70.630458833643,31.2638292832007,201.549999999999));
#24652=CARTESIAN_POINT('',(-101.730458833643,31.263829283201,201.549999999999));
#24653=CARTESIAN_POINT('',(-72.8304588336431,31.2638292832007,204.949999999999));
#24654=CARTESIAN_POINT('',(-72.830458833643,31.2638292832007,198.199999999999));
#24655=CARTESIAN_POINT('',(-70.6304588336431,31.2638292832007,204.949999999999));
#24656=CARTESIAN_POINT('',(-101.730458833643,31.263829283201,204.949999999999));
#24657=CARTESIAN_POINT('',(-70.630458833643,31.2638292832007,198.199999999999));
#24658=CARTESIAN_POINT('',(-76.830458833643,31.2638292832007,201.549999999999));
#24659=CARTESIAN_POINT('',(-74.630458833643,31.2638292832007,201.549999999999));
#24660=CARTESIAN_POINT('',(-101.730458833643,31.263829283201,201.549999999999));
#24661=CARTESIAN_POINT('',(-76.8304588336431,31.2638292832007,204.949999999999));
#24662=CARTESIAN_POINT('',(-76.830458833643,31.2638292832007,198.199999999999));
#24663=CARTESIAN_POINT('',(-74.6304588336431,31.2638292832007,204.949999999999));
#24664=CARTESIAN_POINT('',(-101.730458833643,31.263829283201,204.949999999999));
#24665=CARTESIAN_POINT('',(-74.630458833643,31.2638292832007,198.199999999999));
#24666=CARTESIAN_POINT('',(-80.830458833643,31.2638292832008,201.549999999999));
#24667=CARTESIAN_POINT('',(-78.630458833643,31.2638292832008,201.549999999999));
#24668=CARTESIAN_POINT('',(-101.730458833643,31.263829283201,201.549999999999));
#24669=CARTESIAN_POINT('',(-80.8304588336431,31.2638292832008,204.949999999999));
#24670=CARTESIAN_POINT('',(-80.830458833643,31.2638292832008,198.199999999999));
#24671=CARTESIAN_POINT('',(-78.6304588336431,31.2638292832008,204.949999999999));
#24672=CARTESIAN_POINT('',(-101.730458833643,31.263829283201,204.949999999999));
#24673=CARTESIAN_POINT('',(-78.630458833643,31.2638292832008,198.199999999999));
#24674=CARTESIAN_POINT('',(-84.830458833643,31.2638292832008,201.549999999999));
#24675=CARTESIAN_POINT('',(-82.630458833643,31.2638292832008,201.549999999999));
#24676=CARTESIAN_POINT('',(-101.730458833643,31.263829283201,201.549999999999));
#24677=CARTESIAN_POINT('',(-84.8304588336431,31.2638292832008,204.949999999999));
#24678=CARTESIAN_POINT('',(-84.830458833643,31.2638292832008,198.199999999999));
#24679=CARTESIAN_POINT('',(-82.6304588336431,31.2638292832008,204.949999999999));
#24680=CARTESIAN_POINT('',(-101.730458833643,31.263829283201,204.949999999999));
#24681=CARTESIAN_POINT('',(-82.630458833643,31.2638292832008,198.199999999999));
#24682=CARTESIAN_POINT('',(-82.9804588336431,31.2638292832008,208.749999999999));
#24683=CARTESIAN_POINT('Origin',(-83.7304588336431,31.2638292832008,208.749999999999));
#24684=CARTESIAN_POINT('',(-78.9804588336431,31.2638292832008,208.749999999999));
#24685=CARTESIAN_POINT('Origin',(-79.7304588336431,31.2638292832008,208.749999999999));
#24686=CARTESIAN_POINT('',(-74.9804588336431,31.2638292832007,208.749999999999));
#24687=CARTESIAN_POINT('Origin',(-75.7304588336431,31.2638292832007,208.749999999999));
#24688=CARTESIAN_POINT('',(-70.9804588336431,31.2638292832007,208.749999999999));
#24689=CARTESIAN_POINT('Origin',(-71.7304588336431,31.2638292832007,208.749999999999));
#24690=CARTESIAN_POINT('',(-66.9804588336431,31.2638292832006,208.749999999999));
#24691=CARTESIAN_POINT('Origin',(-67.7304588336431,31.2638292832007,208.749999999999));
#24692=CARTESIAN_POINT('',(-62.9804588336431,31.2638292832006,208.749999999999));
#24693=CARTESIAN_POINT('Origin',(-63.7304588336431,31.2638292832006,208.749999999999));
#24694=CARTESIAN_POINT('',(-58.9804588336431,31.2638292832006,208.749999999999));
#24695=CARTESIAN_POINT('Origin',(-59.7304588336431,31.2638292832006,208.749999999999));
#24696=CARTESIAN_POINT('',(-54.9804588336431,31.2638292832005,208.749999999999));
#24697=CARTESIAN_POINT('Origin',(-55.7304588336431,31.2638292832005,208.749999999999));
#24698=CARTESIAN_POINT('',(-50.9804588336431,31.2638292832005,208.749999999999));
#24699=CARTESIAN_POINT('Origin',(-51.7304588336431,31.2638292832005,208.749999999999));
#24700=CARTESIAN_POINT('',(-46.9804588336431,31.2638292832004,208.75));
#24701=CARTESIAN_POINT('Origin',(-47.7304588336431,31.2638292832005,208.75));
#24702=CARTESIAN_POINT('',(-42.9804588336431,31.2638292832004,208.75));
#24703=CARTESIAN_POINT('Origin',(-43.7304588336431,31.2638292832004,208.75));
#24704=CARTESIAN_POINT('',(-38.9804588336431,31.2638292832004,208.75));
#24705=CARTESIAN_POINT('Origin',(-39.7304588336431,31.2638292832004,208.75));
#24706=CARTESIAN_POINT('',(-34.9804588336431,31.2638292832003,208.75));
#24707=CARTESIAN_POINT('Origin',(-35.7304588336431,31.2638292832003,208.75));
#24708=CARTESIAN_POINT('',(-30.9804588336431,31.2638292832003,208.75));
#24709=CARTESIAN_POINT('Origin',(-31.7304588336431,31.2638292832003,208.75));
#24710=CARTESIAN_POINT('',(-26.9804588336431,31.2638292832002,208.75));
#24711=CARTESIAN_POINT('Origin',(-27.7304588336431,31.2638292832003,208.75));
#24712=CARTESIAN_POINT('',(-22.9804588336431,31.2638292832002,208.75));
#24713=CARTESIAN_POINT('Origin',(-23.7304588336431,31.2638292832002,208.75));
#24714=CARTESIAN_POINT('',(-18.9804588336431,31.2638292832002,208.75));
#24715=CARTESIAN_POINT('Origin',(-19.7304588336431,31.2638292832002,208.75));
#24716=CARTESIAN_POINT('',(-14.9804588336431,31.2638292832001,208.75));
#24717=CARTESIAN_POINT('Origin',(-15.7304588336431,31.2638292832001,208.75));
#24718=CARTESIAN_POINT('',(-10.9804588336431,31.2638292832001,208.75));
#24719=CARTESIAN_POINT('Origin',(-11.7304588336431,31.2638292832001,208.75));
#24720=CARTESIAN_POINT('',(-6.98045883364311,31.2638292832001,208.75));
#24721=CARTESIAN_POINT('Origin',(-7.73045883364311,31.2638292832001,208.75));
#24722=CARTESIAN_POINT('',(-2.9804588336431,31.2638292832,208.75));
#24723=CARTESIAN_POINT('Origin',(-3.7304588336431,31.2638292832,208.75));
#24724=CARTESIAN_POINT('',(1.01954116635688,31.2638292832,208.75));
#24725=CARTESIAN_POINT('Origin',(0.269541166356885,31.2638292832,208.75));
#24726=CARTESIAN_POINT('',(5.01954116635689,31.2638292831999,208.75));
#24727=CARTESIAN_POINT('Origin',(4.26954116635689,31.2638292831999,208.75));
#24728=CARTESIAN_POINT('',(9.01954116635689,31.2638292831999,208.75));
#24729=CARTESIAN_POINT('Origin',(8.26954116635689,31.2638292831999,208.75));
#24730=CARTESIAN_POINT('',(13.0195411663569,31.2638292831998,208.75));
#24731=CARTESIAN_POINT('Origin',(12.2695411663569,31.2638292831999,208.75));
#24732=CARTESIAN_POINT('',(17.0195411663569,31.2638292831998,208.75));
#24733=CARTESIAN_POINT('Origin',(16.2695411663569,31.2638292831998,208.75));
#24734=CARTESIAN_POINT('Origin',(17.369541166357,31.2638292831998,198.2));
#24735=CARTESIAN_POINT('',(17.369541166357,31.2638292831998,201.55));
#24736=CARTESIAN_POINT('',(17.3695411663569,31.2638292831998,204.95));
#24737=CARTESIAN_POINT('Origin',(16.2695411663569,31.2638292831998,208.75));
#24738=CARTESIAN_POINT('',(17.0195411663569,31.2638292831998,208.75));
#24739=CARTESIAN_POINT('Origin',(12.2695411663569,31.2638292831999,208.75));
#24740=CARTESIAN_POINT('',(13.0195411663569,31.2638292831998,208.75));
#24741=CARTESIAN_POINT('Origin',(8.26954116635689,31.2638292831999,208.75));
#24742=CARTESIAN_POINT('',(9.01954116635689,31.2638292831999,208.75));
#24743=CARTESIAN_POINT('Origin',(4.26954116635689,31.2638292831999,208.75));
#24744=CARTESIAN_POINT('',(5.01954116635689,31.2638292831999,208.75));
#24745=CARTESIAN_POINT('Origin',(0.269541166356885,31.2638292832,208.75));
#24746=CARTESIAN_POINT('',(1.01954116635688,31.2638292832,208.75));
#24747=CARTESIAN_POINT('Origin',(-3.7304588336431,31.2638292832,208.75));
#24748=CARTESIAN_POINT('',(-2.9804588336431,31.2638292832,208.75));
#24749=CARTESIAN_POINT('Origin',(-7.73045883364311,31.2638292832001,208.75));
#24750=CARTESIAN_POINT('',(-6.98045883364311,31.2638292832001,208.75));
#24751=CARTESIAN_POINT('Origin',(-11.7304588336431,31.2638292832001,208.75));
#24752=CARTESIAN_POINT('',(-10.9804588336431,31.2638292832001,208.75));
#24753=CARTESIAN_POINT('Origin',(-15.7304588336431,31.2638292832001,208.75));
#24754=CARTESIAN_POINT('',(-14.9804588336431,31.2638292832001,208.75));
#24755=CARTESIAN_POINT('Origin',(-19.7304588336431,31.2638292832002,208.75));
#24756=CARTESIAN_POINT('',(-18.9804588336431,31.2638292832002,208.75));
#24757=CARTESIAN_POINT('Origin',(-23.7304588336431,31.2638292832002,208.75));
#24758=CARTESIAN_POINT('',(-22.9804588336431,31.2638292832002,208.75));
#24759=CARTESIAN_POINT('Origin',(-27.7304588336431,31.2638292832003,208.75));
#24760=CARTESIAN_POINT('',(-26.9804588336431,31.2638292832002,208.75));
#24761=CARTESIAN_POINT('Origin',(-31.7304588336431,31.2638292832003,208.75));
#24762=CARTESIAN_POINT('',(-30.9804588336431,31.2638292832003,208.75));
#24763=CARTESIAN_POINT('Origin',(-35.7304588336431,31.2638292832003,208.75));
#24764=CARTESIAN_POINT('',(-34.9804588336431,31.2638292832003,208.75));
#24765=CARTESIAN_POINT('Origin',(-39.7304588336431,31.2638292832004,208.75));
#24766=CARTESIAN_POINT('',(-38.9804588336431,31.2638292832004,208.75));
#24767=CARTESIAN_POINT('Origin',(-43.7304588336431,31.2638292832004,208.75));
#24768=CARTESIAN_POINT('',(-42.9804588336431,31.2638292832004,208.75));
#24769=CARTESIAN_POINT('Origin',(-47.7304588336431,31.2638292832005,208.75));
#24770=CARTESIAN_POINT('',(-46.9804588336431,31.2638292832004,208.75));
#24771=CARTESIAN_POINT('Origin',(-51.7304588336431,31.2638292832005,208.749999999999));
#24772=CARTESIAN_POINT('',(-50.9804588336431,31.2638292832005,208.749999999999));
#24773=CARTESIAN_POINT('Origin',(-55.7304588336431,31.2638292832005,208.749999999999));
#24774=CARTESIAN_POINT('',(-54.9804588336431,31.2638292832005,208.749999999999));
#24775=CARTESIAN_POINT('Origin',(-59.7304588336431,31.2638292832006,208.749999999999));
#24776=CARTESIAN_POINT('',(-58.9804588336431,31.2638292832006,208.749999999999));
#24777=CARTESIAN_POINT('Origin',(-63.7304588336431,31.2638292832006,208.749999999999));
#24778=CARTESIAN_POINT('',(-62.9804588336431,31.2638292832006,208.749999999999));
#24779=CARTESIAN_POINT('Origin',(-67.7304588336431,31.2638292832007,208.749999999999));
#24780=CARTESIAN_POINT('',(-66.9804588336431,31.2638292832006,208.749999999999));
#24781=CARTESIAN_POINT('Origin',(-71.7304588336431,31.2638292832007,208.749999999999));
#24782=CARTESIAN_POINT('',(-70.9804588336431,31.2638292832007,208.749999999999));
#24783=CARTESIAN_POINT('Origin',(-75.7304588336431,31.2638292832007,208.749999999999));
#24784=CARTESIAN_POINT('',(-74.9804588336431,31.2638292832007,208.749999999999));
#24785=CARTESIAN_POINT('Origin',(-79.7304588336431,31.2638292832008,208.749999999999));
#24786=CARTESIAN_POINT('',(-78.9804588336431,31.2638292832008,208.749999999999));
#24787=CARTESIAN_POINT('Origin',(-83.7304588336431,31.2638292832008,208.749999999999));
#24788=CARTESIAN_POINT('',(-82.9804588336431,31.2638292832008,208.749999999999));
#24789=CARTESIAN_POINT('Origin',(-82.630458833643,31.2638292832008,198.199999999999));
#24790=CARTESIAN_POINT('',(-82.630458833643,31.2638292832008,201.549999999999));
#24791=CARTESIAN_POINT('',(-82.6304588336431,31.2638292832008,204.949999999999));
#24792=CARTESIAN_POINT('Origin',(-78.630458833643,31.2638292832008,198.199999999999));
#24793=CARTESIAN_POINT('',(-78.630458833643,31.2638292832008,201.549999999999));
#24794=CARTESIAN_POINT('',(-78.6304588336431,31.2638292832008,204.949999999999));
#24795=CARTESIAN_POINT('Origin',(-74.630458833643,31.2638292832007,198.199999999999));
#24796=CARTESIAN_POINT('',(-74.630458833643,31.2638292832007,201.549999999999));
#24797=CARTESIAN_POINT('',(-74.6304588336431,31.2638292832007,204.949999999999));
#24798=CARTESIAN_POINT('Origin',(-70.630458833643,31.2638292832007,198.199999999999));
#24799=CARTESIAN_POINT('',(-70.630458833643,31.2638292832007,201.549999999999));
#24800=CARTESIAN_POINT('',(-70.6304588336431,31.2638292832007,204.949999999999));
#24801=CARTESIAN_POINT('Origin',(-66.630458833643,31.2638292832006,198.199999999999));
#24802=CARTESIAN_POINT('',(-66.630458833643,31.2638292832006,201.549999999999));
#24803=CARTESIAN_POINT('',(-66.6304588336431,31.2638292832006,204.949999999999));
#24804=CARTESIAN_POINT('Origin',(-62.630458833643,31.2638292832006,198.199999999999));
#24805=CARTESIAN_POINT('',(-62.6304588336431,31.2638292832006,201.549999999999));
#24806=CARTESIAN_POINT('',(-62.6304588336431,31.2638292832006,204.949999999999));
#24807=CARTESIAN_POINT('Origin',(-58.630458833643,31.2638292832006,198.199999999999));
#24808=CARTESIAN_POINT('',(-58.630458833643,31.2638292832006,201.549999999999));
#24809=CARTESIAN_POINT('',(-58.6304588336431,31.2638292832006,204.949999999999));
#24810=CARTESIAN_POINT('Origin',(-54.630458833643,31.2638292832005,198.199999999999));
#24811=CARTESIAN_POINT('',(-54.630458833643,31.2638292832005,201.549999999999));
#24812=CARTESIAN_POINT('',(-54.6304588336431,31.2638292832005,204.949999999999));
#24813=CARTESIAN_POINT('Origin',(-50.630458833643,31.2638292832005,198.2));
#24814=CARTESIAN_POINT('',(-50.630458833643,31.2638292832005,201.549999999999));
#24815=CARTESIAN_POINT('',(-50.6304588336431,31.2638292832005,204.95));
#24816=CARTESIAN_POINT('Origin',(-46.630458833643,31.2638292832004,198.2));
#24817=CARTESIAN_POINT('',(-46.630458833643,31.2638292832004,201.55));
#24818=CARTESIAN_POINT('',(-46.6304588336431,31.2638292832004,204.95));
#24819=CARTESIAN_POINT('Origin',(-42.630458833643,31.2638292832004,198.2));
#24820=CARTESIAN_POINT('',(-42.630458833643,31.2638292832004,201.55));
#24821=CARTESIAN_POINT('',(-42.6304588336431,31.2638292832004,204.95));
#24822=CARTESIAN_POINT('Origin',(-38.630458833643,31.2638292832004,198.2));
#24823=CARTESIAN_POINT('',(-38.630458833643,31.2638292832004,201.55));
#24824=CARTESIAN_POINT('',(-38.6304588336431,31.2638292832004,204.95));
#24825=CARTESIAN_POINT('Origin',(-34.630458833643,31.2638292832003,198.2));
#24826=CARTESIAN_POINT('',(-34.630458833643,31.2638292832003,201.55));
#24827=CARTESIAN_POINT('',(-34.6304588336431,31.2638292832003,204.95));
#24828=CARTESIAN_POINT('Origin',(-30.630458833643,31.2638292832003,198.2));
#24829=CARTESIAN_POINT('',(-30.630458833643,31.2638292832003,201.55));
#24830=CARTESIAN_POINT('',(-30.6304588336431,31.2638292832003,204.95));
#24831=CARTESIAN_POINT('Origin',(-26.630458833643,31.2638292832002,198.2));
#24832=CARTESIAN_POINT('',(-26.630458833643,31.2638292832002,201.55));
#24833=CARTESIAN_POINT('',(-26.6304588336431,31.2638292832002,204.95));
#24834=CARTESIAN_POINT('Origin',(-22.630458833643,31.2638292832002,198.2));
#24835=CARTESIAN_POINT('',(-22.630458833643,31.2638292832002,201.55));
#24836=CARTESIAN_POINT('',(-22.6304588336431,31.2638292832002,204.95));
#24837=CARTESIAN_POINT('Origin',(-18.630458833643,31.2638292832002,198.2));
#24838=CARTESIAN_POINT('',(-18.630458833643,31.2638292832002,201.55));
#24839=CARTESIAN_POINT('',(-18.6304588336431,31.2638292832002,204.95));
#24840=CARTESIAN_POINT('Origin',(-14.630458833643,31.2638292832001,198.2));
#24841=CARTESIAN_POINT('',(-14.630458833643,31.2638292832001,201.55));
#24842=CARTESIAN_POINT('',(-14.6304588336431,31.2638292832001,204.95));
#24843=CARTESIAN_POINT('Origin',(-10.630458833643,31.2638292832001,198.2));
#24844=CARTESIAN_POINT('',(-10.630458833643,31.2638292832001,201.55));
#24845=CARTESIAN_POINT('',(-10.6304588336431,31.2638292832001,204.95));
#24846=CARTESIAN_POINT('Origin',(-6.63045883364299,31.2638292832,198.2));
#24847=CARTESIAN_POINT('',(-6.63045883364302,31.2638292832,201.55));
#24848=CARTESIAN_POINT('',(-6.63045883364306,31.2638292832,204.95));
#24849=CARTESIAN_POINT('Origin',(-2.630458833643,31.2638292832,198.2));
#24850=CARTESIAN_POINT('',(-2.63045883364303,31.2638292832,201.55));
#24851=CARTESIAN_POINT('',(-2.63045883364307,31.2638292832,204.95));
#24852=CARTESIAN_POINT('Origin',(1.369541166357,31.2638292832,198.2));
#24853=CARTESIAN_POINT('',(1.36954116635697,31.2638292832,201.55));
#24854=CARTESIAN_POINT('',(1.36954116635693,31.2638292832,204.95));
#24855=CARTESIAN_POINT('Origin',(5.369541166357,31.2638292831999,198.2));
#24856=CARTESIAN_POINT('',(5.36954116635698,31.2638292831999,201.55));
#24857=CARTESIAN_POINT('',(5.36954116635693,31.2638292831999,204.95));
#24858=CARTESIAN_POINT('Origin',(9.36954116635701,31.2638292831999,198.2));
#24859=CARTESIAN_POINT('',(9.36954116635698,31.2638292831999,201.55));
#24860=CARTESIAN_POINT('',(9.36954116635694,31.2638292831999,204.95));
#24861=CARTESIAN_POINT('Origin',(13.369541166357,31.2638292831998,198.2));
#24862=CARTESIAN_POINT('',(13.369541166357,31.2638292831998,201.55));
#24863=CARTESIAN_POINT('',(13.3695411663569,31.2638292831998,204.95));
#24864=CARTESIAN_POINT('Origin',(-101.730458833643,31.263829283201,210.499999999999));
#24865=CARTESIAN_POINT('',(-85.6069914720345,31.2638292832008,210.499999999999));
#24866=CARTESIAN_POINT('',(18.2695411663569,31.2638292831998,210.5));
#24867=CARTESIAN_POINT('Origin',(18.269541166357,31.2638292831998,198.2));
#24868=CARTESIAN_POINT('',(18.269541166357,31.2638292831998,198.2));
#24869=CARTESIAN_POINT('Origin',(-101.730458833643,31.263829283201,198.199999999999));
#24870=CARTESIAN_POINT('',(-85.6069914720345,31.2638292832008,198.199999999999));
#24871=CARTESIAN_POINT('Origin',(-101.730458833643,31.263829283201,204.949999999999));
#24872=CARTESIAN_POINT('',(-84.8304588336431,31.2638292832008,204.949999999999));
#24873=CARTESIAN_POINT('Origin',(-84.830458833643,31.2638292832008,198.199999999999));
#24874=CARTESIAN_POINT('',(-84.830458833643,31.2638292832008,201.549999999999));
#24875=CARTESIAN_POINT('Origin',(-101.730458833643,31.263829283201,201.549999999999));
#24876=CARTESIAN_POINT('Origin',(-101.730458833643,31.263829283201,204.949999999999));
#24877=CARTESIAN_POINT('',(-80.8304588336431,31.2638292832008,204.949999999999));
#24878=CARTESIAN_POINT('Origin',(-80.830458833643,31.2638292832008,198.199999999999));
#24879=CARTESIAN_POINT('',(-80.830458833643,31.2638292832008,201.549999999999));
#24880=CARTESIAN_POINT('Origin',(-101.730458833643,31.263829283201,201.549999999999));
#24881=CARTESIAN_POINT('Origin',(-101.730458833643,31.263829283201,204.949999999999));
#24882=CARTESIAN_POINT('',(-76.8304588336431,31.2638292832007,204.949999999999));
#24883=CARTESIAN_POINT('Origin',(-76.830458833643,31.2638292832007,198.199999999999));
#24884=CARTESIAN_POINT('',(-76.830458833643,31.2638292832007,201.549999999999));
#24885=CARTESIAN_POINT('Origin',(-101.730458833643,31.263829283201,201.549999999999));
#24886=CARTESIAN_POINT('Origin',(-101.730458833643,31.263829283201,204.949999999999));
#24887=CARTESIAN_POINT('',(-72.8304588336431,31.2638292832007,204.949999999999));
#24888=CARTESIAN_POINT('Origin',(-72.830458833643,31.2638292832007,198.199999999999));
#24889=CARTESIAN_POINT('',(-72.830458833643,31.2638292832007,201.549999999999));
#24890=CARTESIAN_POINT('Origin',(-101.730458833643,31.263829283201,201.549999999999));
#24891=CARTESIAN_POINT('Origin',(-101.730458833643,31.263829283201,204.949999999999));
#24892=CARTESIAN_POINT('',(-68.8304588336431,31.2638292832007,204.949999999999));
#24893=CARTESIAN_POINT('Origin',(-68.830458833643,31.2638292832007,198.199999999999));
#24894=CARTESIAN_POINT('',(-68.830458833643,31.2638292832007,201.549999999999));
#24895=CARTESIAN_POINT('Origin',(-101.730458833643,31.263829283201,201.549999999999));
#24896=CARTESIAN_POINT('Origin',(-101.730458833643,31.263829283201,204.949999999999));
#24897=CARTESIAN_POINT('',(-64.8304588336431,31.2638292832006,204.949999999999));
#24898=CARTESIAN_POINT('Origin',(-64.830458833643,31.2638292832006,198.199999999999));
#24899=CARTESIAN_POINT('',(-64.830458833643,31.2638292832006,201.549999999999));
#24900=CARTESIAN_POINT('Origin',(-101.730458833643,31.263829283201,201.549999999999));
#24901=CARTESIAN_POINT('Origin',(-101.730458833643,31.263829283201,204.949999999999));
#24902=CARTESIAN_POINT('',(-60.8304588336431,31.2638292832006,204.949999999999));
#24903=CARTESIAN_POINT('Origin',(-60.830458833643,31.2638292832006,198.199999999999));
#24904=CARTESIAN_POINT('',(-60.830458833643,31.2638292832006,201.549999999999));
#24905=CARTESIAN_POINT('Origin',(-101.730458833643,31.263829283201,201.549999999999));
#24906=CARTESIAN_POINT('Origin',(-101.730458833643,31.263829283201,204.949999999999));
#24907=CARTESIAN_POINT('',(-56.8304588336431,31.2638292832006,204.949999999999));
#24908=CARTESIAN_POINT('Origin',(-56.830458833643,31.2638292832006,198.199999999999));
#24909=CARTESIAN_POINT('',(-56.830458833643,31.2638292832006,201.549999999999));
#24910=CARTESIAN_POINT('Origin',(-101.730458833643,31.263829283201,201.549999999999));
#24911=CARTESIAN_POINT('Origin',(-101.730458833643,31.263829283201,204.949999999999));
#24912=CARTESIAN_POINT('',(-52.8304588336431,31.2638292832005,204.949999999999));
#24913=CARTESIAN_POINT('Origin',(-52.830458833643,31.2638292832005,198.2));
#24914=CARTESIAN_POINT('',(-52.830458833643,31.2638292832005,201.549999999999));
#24915=CARTESIAN_POINT('Origin',(-101.730458833643,31.263829283201,201.549999999999));
#24916=CARTESIAN_POINT('Origin',(-101.730458833643,31.263829283201,204.949999999999));
#24917=CARTESIAN_POINT('',(-48.8304588336431,31.2638292832005,204.95));
#24918=CARTESIAN_POINT('Origin',(-48.830458833643,31.2638292832005,198.2));
#24919=CARTESIAN_POINT('',(-48.830458833643,31.2638292832005,201.549999999999));
#24920=CARTESIAN_POINT('Origin',(-101.730458833643,31.263829283201,201.549999999999));
#24921=CARTESIAN_POINT('Origin',(-101.730458833643,31.263829283201,204.949999999999));
#24922=CARTESIAN_POINT('',(-44.8304588336431,31.2638292832004,204.95));
#24923=CARTESIAN_POINT('Origin',(-44.830458833643,31.2638292832004,198.2));
#24924=CARTESIAN_POINT('',(-44.830458833643,31.2638292832004,201.55));
#24925=CARTESIAN_POINT('Origin',(-101.730458833643,31.263829283201,201.549999999999));
#24926=CARTESIAN_POINT('Origin',(-101.730458833643,31.263829283201,204.949999999999));
#24927=CARTESIAN_POINT('',(-40.8304588336431,31.2638292832004,204.95));
#24928=CARTESIAN_POINT('Origin',(-40.830458833643,31.2638292832004,198.2));
#24929=CARTESIAN_POINT('',(-40.830458833643,31.2638292832004,201.55));
#24930=CARTESIAN_POINT('Origin',(-101.730458833643,31.263829283201,201.549999999999));
#24931=CARTESIAN_POINT('Origin',(-101.730458833643,31.263829283201,204.949999999999));
#24932=CARTESIAN_POINT('',(-36.8304588336431,31.2638292832004,204.95));
#24933=CARTESIAN_POINT('Origin',(-36.830458833643,31.2638292832004,198.2));
#24934=CARTESIAN_POINT('',(-36.830458833643,31.2638292832004,201.55));
#24935=CARTESIAN_POINT('Origin',(-101.730458833643,31.263829283201,201.549999999999));
#24936=CARTESIAN_POINT('Origin',(-101.730458833643,31.263829283201,204.949999999999));
#24937=CARTESIAN_POINT('',(-32.8304588336431,31.2638292832003,204.95));
#24938=CARTESIAN_POINT('Origin',(-32.830458833643,31.2638292832003,198.2));
#24939=CARTESIAN_POINT('',(-32.830458833643,31.2638292832003,201.55));
#24940=CARTESIAN_POINT('Origin',(-101.730458833643,31.263829283201,201.549999999999));
#24941=CARTESIAN_POINT('Origin',(-101.730458833643,31.263829283201,204.949999999999));
#24942=CARTESIAN_POINT('',(-28.8304588336431,31.2638292832003,204.95));
#24943=CARTESIAN_POINT('Origin',(-28.830458833643,31.2638292832003,198.2));
#24944=CARTESIAN_POINT('',(-28.830458833643,31.2638292832003,201.55));
#24945=CARTESIAN_POINT('Origin',(-101.730458833643,31.263829283201,201.549999999999));
#24946=CARTESIAN_POINT('Origin',(-101.730458833643,31.263829283201,204.949999999999));
#24947=CARTESIAN_POINT('',(-24.8304588336431,31.2638292832002,204.95));
#24948=CARTESIAN_POINT('Origin',(-24.830458833643,31.2638292832002,198.2));
#24949=CARTESIAN_POINT('',(-24.830458833643,31.2638292832002,201.55));
#24950=CARTESIAN_POINT('Origin',(-101.730458833643,31.263829283201,201.549999999999));
#24951=CARTESIAN_POINT('Origin',(-101.730458833643,31.263829283201,204.949999999999));
#24952=CARTESIAN_POINT('',(-20.8304588336431,31.2638292832002,204.95));
#24953=CARTESIAN_POINT('Origin',(-20.830458833643,31.2638292832002,198.2));
#24954=CARTESIAN_POINT('',(-20.830458833643,31.2638292832002,201.55));
#24955=CARTESIAN_POINT('Origin',(-101.730458833643,31.263829283201,201.549999999999));
#24956=CARTESIAN_POINT('Origin',(-101.730458833643,31.263829283201,204.949999999999));
#24957=CARTESIAN_POINT('',(-16.8304588336431,31.2638292832002,204.95));
#24958=CARTESIAN_POINT('Origin',(-16.830458833643,31.2638292832002,198.2));
#24959=CARTESIAN_POINT('',(-16.830458833643,31.2638292832002,201.55));
#24960=CARTESIAN_POINT('Origin',(-101.730458833643,31.263829283201,201.549999999999));
#24961=CARTESIAN_POINT('Origin',(-101.730458833643,31.263829283201,204.949999999999));
#24962=CARTESIAN_POINT('',(-12.8304588336431,31.2638292832001,204.95));
#24963=CARTESIAN_POINT('Origin',(-12.830458833643,31.2638292832001,198.2));
#24964=CARTESIAN_POINT('',(-12.830458833643,31.2638292832001,201.55));
#24965=CARTESIAN_POINT('Origin',(-101.730458833643,31.263829283201,201.549999999999));
#24966=CARTESIAN_POINT('Origin',(-101.730458833643,31.263829283201,204.949999999999));
#24967=CARTESIAN_POINT('',(-8.83045883364307,31.2638292832001,204.95));
#24968=CARTESIAN_POINT('Origin',(-8.830458833643,31.2638292832001,198.2));
#24969=CARTESIAN_POINT('',(-8.83045883364303,31.2638292832001,201.55));
#24970=CARTESIAN_POINT('Origin',(-101.730458833643,31.263829283201,201.549999999999));
#24971=CARTESIAN_POINT('Origin',(-101.730458833643,31.263829283201,204.949999999999));
#24972=CARTESIAN_POINT('',(-4.83045883364307,31.2638292832,204.95));
#24973=CARTESIAN_POINT('Origin',(-4.830458833643,31.2638292832,198.2));
#24974=CARTESIAN_POINT('',(-4.83045883364302,31.2638292832,201.55));
#24975=CARTESIAN_POINT('Origin',(-101.730458833643,31.263829283201,201.549999999999));
#24976=CARTESIAN_POINT('Origin',(-101.730458833643,31.263829283201,204.949999999999));
#24977=CARTESIAN_POINT('',(-0.830458833643063,31.2638292832,204.95));
#24978=CARTESIAN_POINT('Origin',(-0.830458833642994,31.2638292832,198.2));
#24979=CARTESIAN_POINT('',(-0.830458833643022,31.2638292832,201.55));
#24980=CARTESIAN_POINT('Origin',(-101.730458833643,31.263829283201,201.549999999999));
#24981=CARTESIAN_POINT('Origin',(-101.730458833643,31.263829283201,204.949999999999));
#24982=CARTESIAN_POINT('',(3.16954116635693,31.2638292832,204.95));
#24983=CARTESIAN_POINT('Origin',(3.169541166357,31.2638292832,198.2));
#24984=CARTESIAN_POINT('',(3.16954116635697,31.2638292832,201.55));
#24985=CARTESIAN_POINT('Origin',(-101.730458833643,31.263829283201,201.549999999999));
#24986=CARTESIAN_POINT('Origin',(-101.730458833643,31.263829283201,204.949999999999));
#24987=CARTESIAN_POINT('',(7.16954116635693,31.2638292831999,204.95));
#24988=CARTESIAN_POINT('Origin',(7.169541166357,31.2638292831999,198.2));
#24989=CARTESIAN_POINT('',(7.16954116635697,31.2638292831999,201.55));
#24990=CARTESIAN_POINT('Origin',(-101.730458833643,31.263829283201,201.549999999999));
#24991=CARTESIAN_POINT('Origin',(-101.730458833643,31.263829283201,204.949999999999));
#24992=CARTESIAN_POINT('',(11.1695411663569,31.2638292831999,204.95));
#24993=CARTESIAN_POINT('Origin',(11.169541166357,31.2638292831999,198.2));
#24994=CARTESIAN_POINT('',(11.169541166357,31.2638292831999,201.55));
#24995=CARTESIAN_POINT('Origin',(-101.730458833643,31.263829283201,201.549999999999));
#24996=CARTESIAN_POINT('Origin',(-101.730458833643,31.263829283201,204.949999999999));
#24997=CARTESIAN_POINT('',(15.1695411663569,31.2638292831998,204.95));
#24998=CARTESIAN_POINT('Origin',(15.169541166357,31.2638292831998,198.2));
#24999=CARTESIAN_POINT('',(15.169541166357,31.2638292831998,201.55));
#25000=CARTESIAN_POINT('Origin',(-101.730458833643,31.263829283201,201.549999999999));
#25001=CARTESIAN_POINT('Origin',(-85.6069914720347,10.7638292832008,194.611133062546));
#36646=UNCERTAINTY_MEASURE_WITH_UNIT(LENGTH_MEASURE(0.01),#36669,
'DISTANCE_ACCURACY_VALUE',
'Maximum model space distance between geometric entities at asserted c
onnectivities');
#36656=UNCERTAINTY_MEASURE_WITH_UNIT(LENGTH_MEASURE(0.01),#36669,
'DISTANCE_ACCURACY_VALUE',
'Maximum model space distance between geometric entities at asserted c
onnectivities');
#36658=(
GEOMETRIC_REPRESENTATION_CONTEXT(3)
GLOBAL_UNCERTAINTY_ASSIGNED_CONTEXT((#36646))
GLOBAL_UNIT_ASSIGNED_CONTEXT((#36669,#36671,#36672))
REPRESENTATION_CONTEXT('','3D')
);
#36668=(
GEOMETRIC_REPRESENTATION_CONTEXT(3)
GLOBAL_UNCERTAINTY_ASSIGNED_CONTEXT((#36656))
GLOBAL_UNIT_ASSIGNED_CONTEXT((#36669,#36671,#36672))
REPRESENTATION_CONTEXT('','3D')
);
#36669=(
LENGTH_UNIT()
NAMED_UNIT(*)
SI_UNIT(.MILLI.,.METRE.)
);
#36671=(
NAMED_UNIT(*)
PLANE_ANGLE_UNIT()
SI_UNIT($,.RADIAN.)
);
#36672=(
NAMED_UNIT(*)
SI_UNIT($,.STERADIAN.)
SOLID_ANGLE_UNIT()
);
#36674=SHAPE_DEFINITION_REPRESENTATION(#36685,#36706);
#36685=PRODUCT_DEFINITION_SHAPE('',$,#36718);
#36706=SHAPE_REPRESENTATION('',(#17916),#36658);
#36716=PRODUCT_DEFINITION_CONTEXT('part definition',#36751,'design');
#36718=PRODUCT_DEFINITION('Tape','Tape',#36729,#36716);
#36729=PRODUCT_DEFINITION_FORMATION('',$,#36754);
#36751=APPLICATION_CONTEXT(
'Core Data for Automotive Mechanical Design Process');
#36752=PRODUCT_CONTEXT('part definition',#36751,'mechanical');
#36754=PRODUCT('Tape','Tape',$,(#36752));
#36765=PRESENTATION_STYLE_ASSIGNMENT((#36772));
#36772=SURFACE_STYLE_USAGE(.BOTH.,#36779);
#36779=SURFACE_SIDE_STYLE('',(#36786));
#36786=SURFACE_STYLE_FILL_AREA(#36793);
#36793=FILL_AREA_STYLE('Opaque(23,69,131)',(#36800));
#36800=FILL_AREA_STYLE_COLOUR('Opaque(23,69,131)',#36807);
#36807=COLOUR_RGB('Opaque(23,69,131)',0.0901960784313725,0.270588235294118,
0.513725490196078);
ENDSEC;
END-ISO-10303-21;
